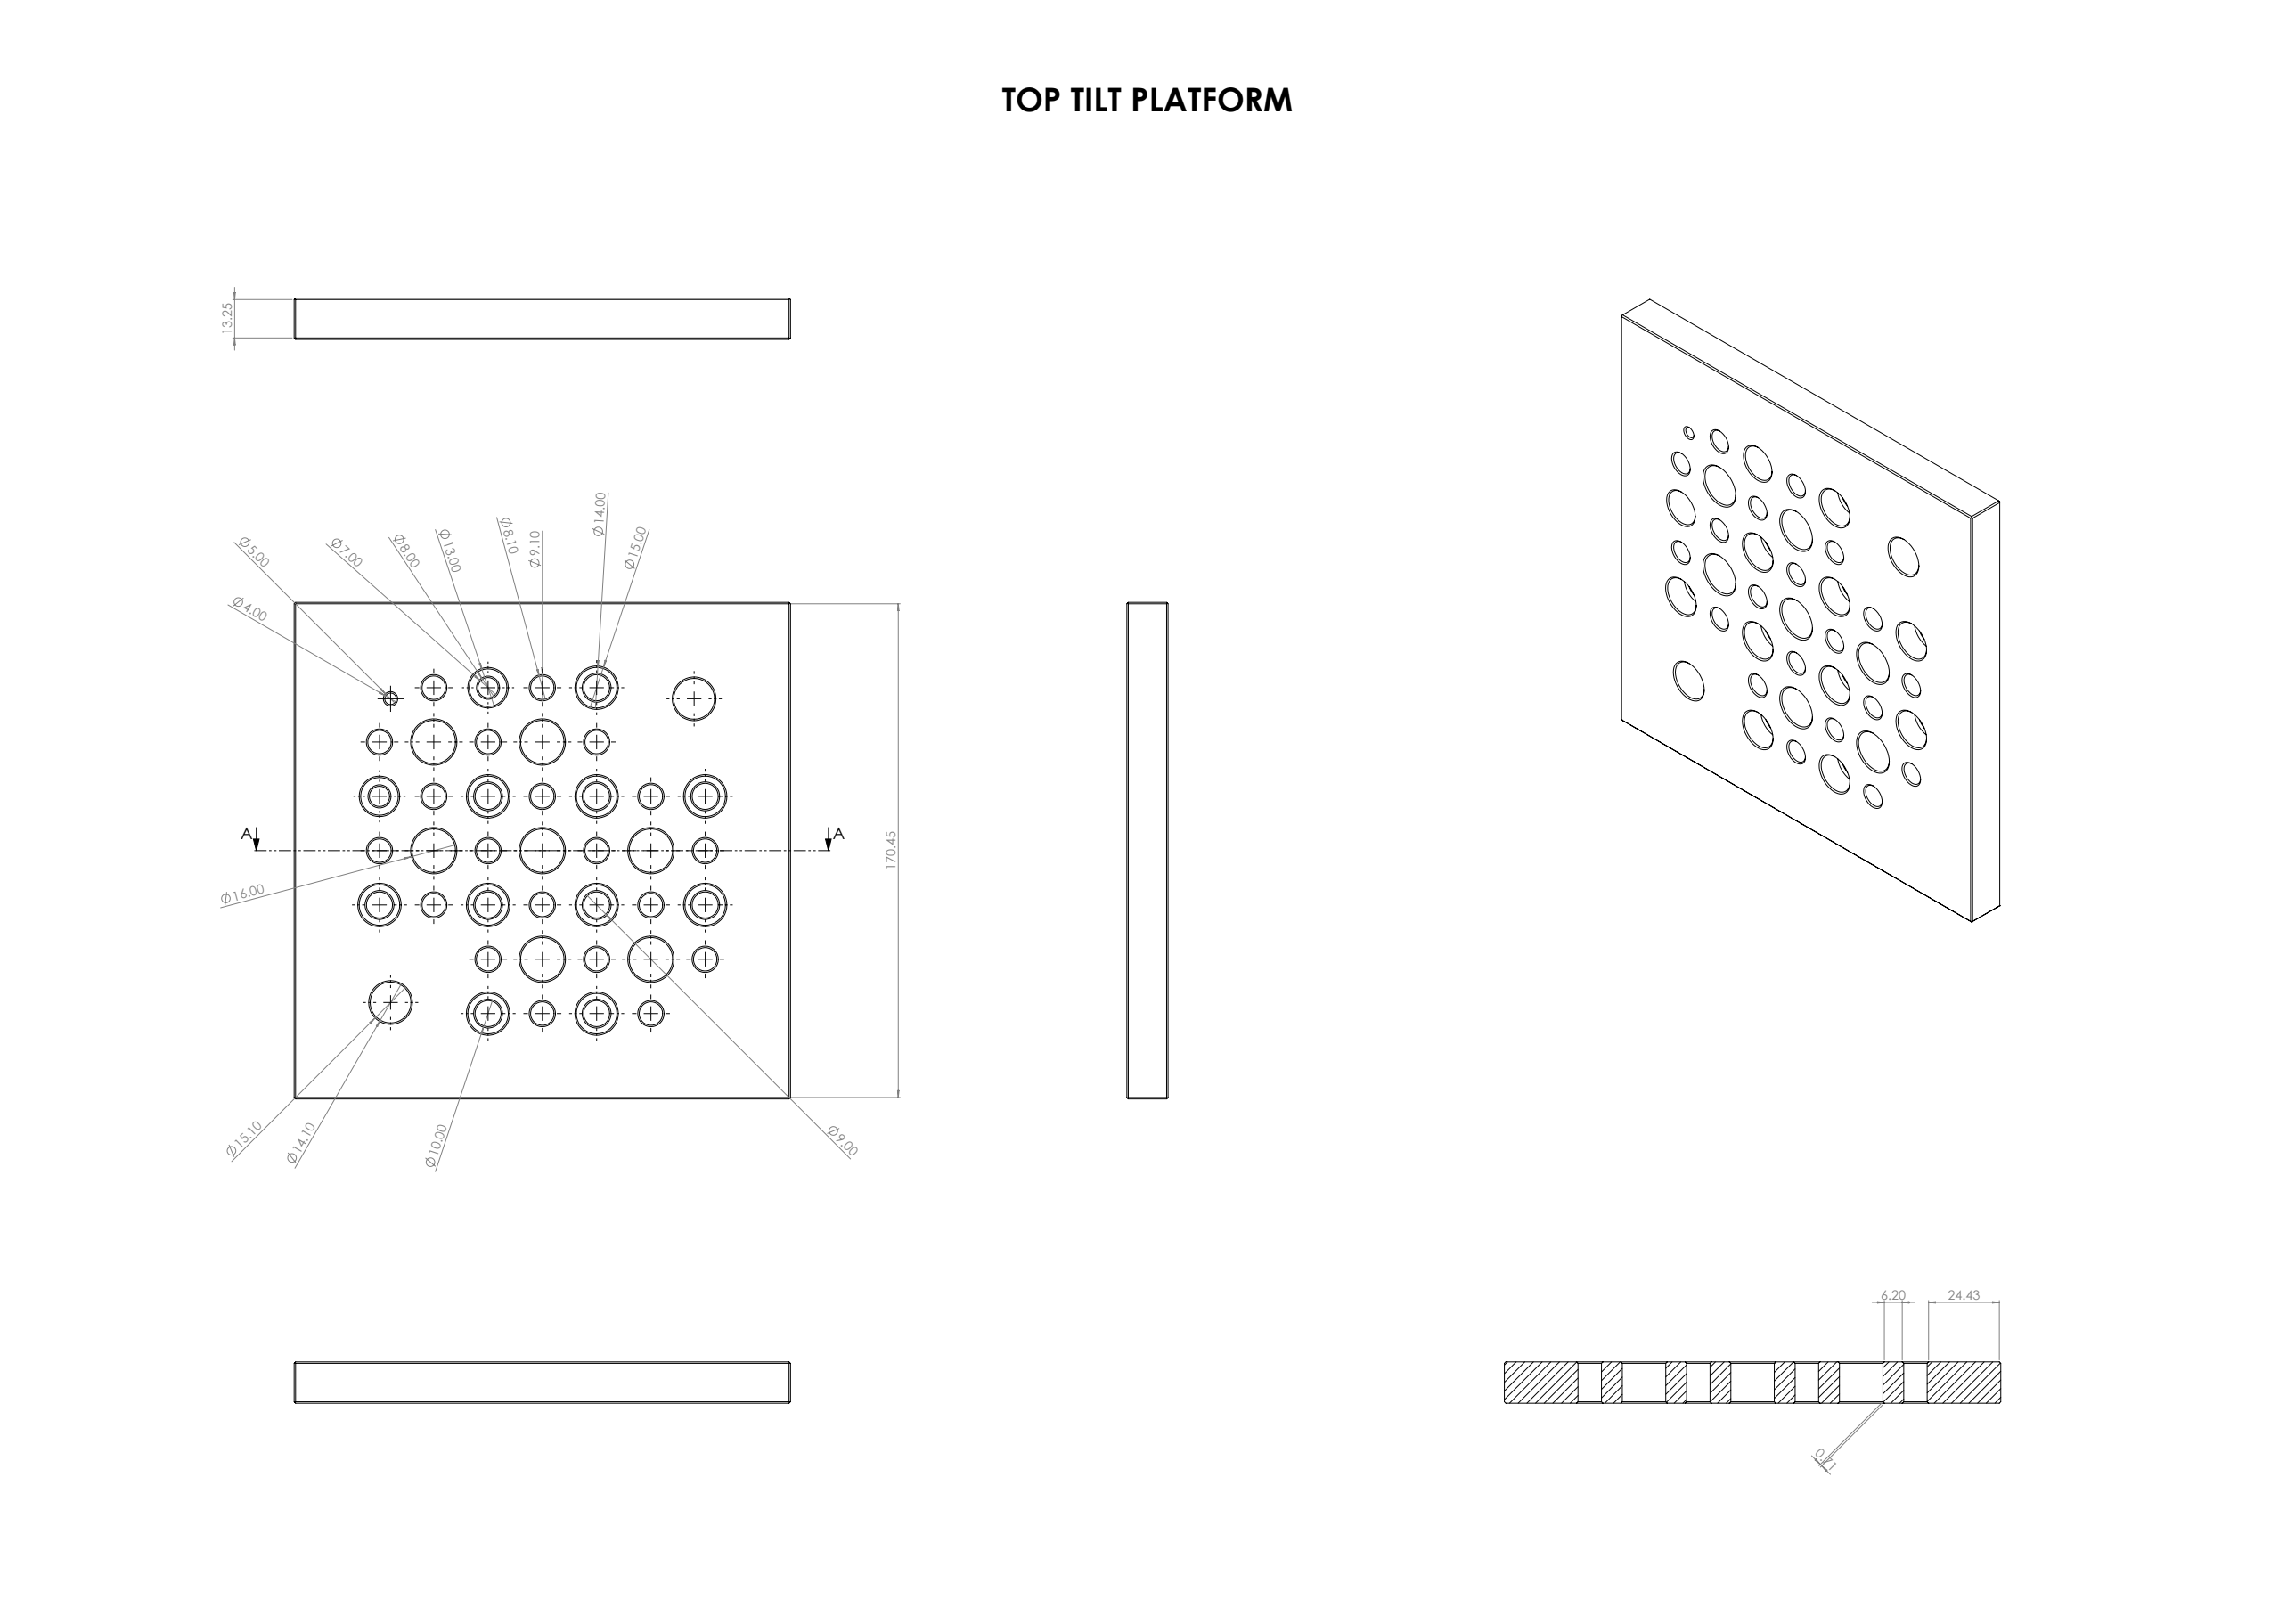
ISO-10303-21;
HEADER;
/* Generated by software containing ST-Developer
 * from STEP Tools, Inc. (www.steptools.com) 
 */

FILE_DESCRIPTION(
/* description */ (''),
/* implementation_level */ '2;1');

FILE_NAME(
/* name */ '03_Top_Tilt_Platform.step',
/* time_stamp */ '2026-10-21T01:56:51-07:00',
/* author */ (''),
/* organization */ (''),
/* preprocessor_version */ 'ST-DEVELOPER v20.2',
/* originating_system */ 'Autodesk Translation Framework v15.15.0.0',
/* authorisation */ '');

FILE_SCHEMA (('AUTOMOTIVE_DESIGN { 1 0 10303 214 3 1 1 }'));
ENDSEC;

DATA;
#10=MECHANICAL_DESIGN_GEOMETRIC_PRESENTATION_REPRESENTATION('',(#272),#82384);
#234=SHAPE_REPRESENTATION_RELATIONSHIP('SRR','None',#82468,#253);
#253=ADVANCED_BREP_SHAPE_REPRESENTATION('',(#291),#82367);
#272=STYLED_ITEM('',(#82645),#291);
#291=MANIFOLD_SOLID_BREP('Body1',#30663);
#483=CYLINDRICAL_SURFACE('',#31325,4.5);
#484=CYLINDRICAL_SURFACE('',#31332,4.5);
#485=CYLINDRICAL_SURFACE('',#31339,4.5);
#486=CYLINDRICAL_SURFACE('',#31346,4.5);
#487=CYLINDRICAL_SURFACE('',#31353,4.5);
#488=CYLINDRICAL_SURFACE('',#31360,4.5);
#489=CYLINDRICAL_SURFACE('',#31367,4.5);
#490=CYLINDRICAL_SURFACE('',#31374,4.5);
#491=CYLINDRICAL_SURFACE('',#31381,2.);
#492=CYLINDRICAL_SURFACE('',#31392,3.5);
#493=CYLINDRICAL_SURFACE('',#31399,3.5);
#494=CYLINDRICAL_SURFACE('',#31412,4.5);
#495=CYLINDRICAL_SURFACE('',#31419,4.5);
#496=CYLINDRICAL_SURFACE('',#31476,7.05);
#497=CYLINDRICAL_SURFACE('',#31480,7.05);
#498=CYLINDRICAL_SURFACE('',#31489,4.05);
#499=CYLINDRICAL_SURFACE('',#31493,4.05);
#500=CYLINDRICAL_SURFACE('',#31497,4.05);
#501=CYLINDRICAL_SURFACE('',#31501,4.05);
#502=CYLINDRICAL_SURFACE('',#31505,4.05);
#503=CYLINDRICAL_SURFACE('',#31509,4.05);
#504=CYLINDRICAL_SURFACE('',#31513,4.05);
#505=CYLINDRICAL_SURFACE('',#31517,4.05);
#506=CYLINDRICAL_SURFACE('',#31521,4.05);
#507=CYLINDRICAL_SURFACE('',#31525,4.05);
#508=CYLINDRICAL_SURFACE('',#31529,4.05);
#509=CYLINDRICAL_SURFACE('',#31533,4.05);
#510=CYLINDRICAL_SURFACE('',#31539,4.05);
#511=CYLINDRICAL_SURFACE('',#31543,4.05);
#512=CYLINDRICAL_SURFACE('',#31547,4.05);
#513=CYLINDRICAL_SURFACE('',#31551,4.05);
#514=CYLINDRICAL_SURFACE('',#31555,4.05);
#515=CYLINDRICAL_SURFACE('',#31559,4.05);
#516=CYLINDRICAL_SURFACE('',#31563,4.05);
#517=CYLINDRICAL_SURFACE('',#31567,4.05);
#518=CYLINDRICAL_SURFACE('',#31571,7.5);
#519=CYLINDRICAL_SURFACE('',#31575,7.5);
#520=CYLINDRICAL_SURFACE('',#31579,7.5);
#521=CYLINDRICAL_SURFACE('',#31583,7.5);
#522=CYLINDRICAL_SURFACE('',#31587,7.5);
#523=CYLINDRICAL_SURFACE('',#31591,7.5);
#524=CYLINDRICAL_SURFACE('',#31595,7.5);
#525=CYLINDRICAL_SURFACE('',#31652,7.);
#526=CYLINDRICAL_SURFACE('',#31655,7.);
#527=CYLINDRICAL_SURFACE('',#31658,7.);
#528=CYLINDRICAL_SURFACE('',#31661,7.);
#529=CYLINDRICAL_SURFACE('',#31664,7.);
#530=CYLINDRICAL_SURFACE('',#31667,7.);
#531=CYLINDRICAL_SURFACE('',#31670,7.);
#532=CYLINDRICAL_SURFACE('',#31673,7.);
#533=CYLINDRICAL_SURFACE('',#31676,7.);
#534=CYLINDRICAL_SURFACE('',#31679,7.);
#535=CYLINDRICAL_SURFACE('',#31704,6.5);
#536=CYLINDRICAL_SURFACE('',#31707,6.5);
#537=CYLINDRICAL_SURFACE('',#31708,4.2379);
#1196=CIRCLE('',#31323,4.5);
#1197=CIRCLE('',#31324,5.);
#1198=CIRCLE('',#31326,4.5);
#1199=CIRCLE('',#31328,7.);
#1200=CIRCLE('',#31330,4.5);
#1201=CIRCLE('',#31331,5.);
#1202=CIRCLE('',#31333,4.5);
#1203=CIRCLE('',#31335,7.);
#1204=CIRCLE('',#31337,4.5);
#1205=CIRCLE('',#31338,5.);
#1206=CIRCLE('',#31340,4.5);
#1207=CIRCLE('',#31342,7.);
#1208=CIRCLE('',#31344,4.5);
#1209=CIRCLE('',#31345,5.);
#1210=CIRCLE('',#31347,4.5);
#1211=CIRCLE('',#31349,7.);
#1212=CIRCLE('',#31351,4.5);
#1213=CIRCLE('',#31352,5.);
#1214=CIRCLE('',#31354,4.5);
#1215=CIRCLE('',#31356,7.);
#1216=CIRCLE('',#31358,4.5);
#1217=CIRCLE('',#31359,5.);
#1218=CIRCLE('',#31361,4.5);
#1219=CIRCLE('',#31363,7.);
#1220=CIRCLE('',#31365,4.5);
#1221=CIRCLE('',#31366,5.);
#1222=CIRCLE('',#31368,4.5);
#1223=CIRCLE('',#31370,7.);
#1224=CIRCLE('',#31372,4.5);
#1225=CIRCLE('',#31373,5.);
#1226=CIRCLE('',#31375,4.5);
#1227=CIRCLE('',#31377,7.);
#1228=CIRCLE('',#31379,2.);
#1229=CIRCLE('',#31380,2.5);
#1230=CIRCLE('',#31382,2.);
#1231=CIRCLE('',#31384,4.2379);
#1232=CIRCLE('',#31390,3.5);
#1233=CIRCLE('',#31391,4.);
#1234=CIRCLE('',#31393,3.5);
#1235=CIRCLE('',#31395,6.5);
#1236=CIRCLE('',#31397,3.5);
#1237=CIRCLE('',#31398,3.99999999999999);
#1238=CIRCLE('',#31400,3.5);
#1239=CIRCLE('',#31402,6.5);
#1240=CIRCLE('',#31410,4.5);
#1241=CIRCLE('',#31411,5.);
#1242=CIRCLE('',#31413,4.5);
#1243=CIRCLE('',#31415,7.);
#1244=CIRCLE('',#31417,4.5);
#1245=CIRCLE('',#31418,5.);
#1246=CIRCLE('',#31420,4.5);
#1247=CIRCLE('',#31422,7.);
#1248=CIRCLE('',#31424,5.);
#1249=CIRCLE('',#31426,5.);
#1250=CIRCLE('',#31427,5.);
#1251=CIRCLE('',#31428,5.);
#1252=CIRCLE('',#31429,5.);
#1253=CIRCLE('',#31430,7.55);
#1254=CIRCLE('',#31431,5.);
#1255=CIRCLE('',#31432,4.55);
#1256=CIRCLE('',#31433,4.55);
#1257=CIRCLE('',#31434,4.55);
#1258=CIRCLE('',#31435,4.55);
#1259=CIRCLE('',#31436,4.55);
#1260=CIRCLE('',#31437,4.55);
#1261=CIRCLE('',#31438,3.99999999999999);
#1262=CIRCLE('',#31439,4.55);
#1263=CIRCLE('',#31440,4.55);
#1264=CIRCLE('',#31441,4.55);
#1265=CIRCLE('',#31442,4.55);
#1266=CIRCLE('',#31443,8.);
#1267=CIRCLE('',#31444,8.);
#1268=CIRCLE('',#31445,8.);
#1269=CIRCLE('',#31446,8.);
#1270=CIRCLE('',#31447,4.2379);
#1271=CIRCLE('',#31448,8.);
#1272=CIRCLE('',#31449,8.);
#1273=CIRCLE('',#31450,8.);
#1274=CIRCLE('',#31451,4.55);
#1275=CIRCLE('',#31452,4.55);
#1276=CIRCLE('',#31453,4.55);
#1277=CIRCLE('',#31454,4.55);
#1278=CIRCLE('',#31455,4.);
#1279=CIRCLE('',#31456,4.55);
#1280=CIRCLE('',#31457,4.55);
#1281=CIRCLE('',#31458,4.55);
#1282=CIRCLE('',#31459,4.55);
#1283=CIRCLE('',#31460,4.55);
#1284=CIRCLE('',#31461,4.55);
#1285=CIRCLE('',#31462,5.);
#1286=CIRCLE('',#31463,7.55);
#1287=CIRCLE('',#31464,5.);
#1288=CIRCLE('',#31465,5.);
#1289=CIRCLE('',#31466,5.);
#1290=CIRCLE('',#31475,7.05);
#1291=CIRCLE('',#31477,7.05);
#1292=CIRCLE('',#31479,7.05);
#1293=CIRCLE('',#31481,7.05);
#1294=CIRCLE('',#31488,4.05);
#1295=CIRCLE('',#31490,4.05);
#1296=CIRCLE('',#31492,4.05);
#1297=CIRCLE('',#31494,4.05);
#1298=CIRCLE('',#31496,4.05);
#1299=CIRCLE('',#31498,4.05);
#1300=CIRCLE('',#31500,4.05);
#1301=CIRCLE('',#31502,4.05);
#1302=CIRCLE('',#31504,4.05);
#1303=CIRCLE('',#31506,4.05);
#1304=CIRCLE('',#31508,4.05);
#1305=CIRCLE('',#31510,4.05);
#1306=CIRCLE('',#31512,4.05);
#1307=CIRCLE('',#31514,4.05);
#1308=CIRCLE('',#31516,4.05);
#1309=CIRCLE('',#31518,4.05);
#1310=CIRCLE('',#31520,4.05);
#1311=CIRCLE('',#31522,4.05);
#1312=CIRCLE('',#31524,4.05);
#1313=CIRCLE('',#31526,4.05);
#1314=CIRCLE('',#31528,4.05);
#1315=CIRCLE('',#31530,4.05);
#1316=CIRCLE('',#31532,4.05);
#1317=CIRCLE('',#31534,4.05);
#1318=CIRCLE('',#31538,4.05);
#1319=CIRCLE('',#31540,4.05);
#1320=CIRCLE('',#31542,4.05);
#1321=CIRCLE('',#31544,4.05);
#1322=CIRCLE('',#31546,4.05);
#1323=CIRCLE('',#31548,4.05);
#1324=CIRCLE('',#31550,4.05);
#1325=CIRCLE('',#31552,4.05);
#1326=CIRCLE('',#31554,4.05);
#1327=CIRCLE('',#31556,4.05);
#1328=CIRCLE('',#31558,4.05);
#1329=CIRCLE('',#31560,4.05);
#1330=CIRCLE('',#31562,4.05);
#1331=CIRCLE('',#31564,4.05);
#1332=CIRCLE('',#31566,4.05);
#1333=CIRCLE('',#31568,4.05);
#1334=CIRCLE('',#31570,7.5);
#1335=CIRCLE('',#31572,7.5);
#1336=CIRCLE('',#31574,7.5);
#1337=CIRCLE('',#31576,7.5);
#1338=CIRCLE('',#31578,7.5);
#1339=CIRCLE('',#31580,7.5);
#1340=CIRCLE('',#31582,7.5);
#1341=CIRCLE('',#31584,7.5);
#1342=CIRCLE('',#31586,7.5);
#1343=CIRCLE('',#31588,7.5);
#1344=CIRCLE('',#31590,7.5);
#1345=CIRCLE('',#31592,7.5);
#1346=CIRCLE('',#31594,7.5);
#1347=CIRCLE('',#31596,7.5);
#1348=CIRCLE('',#31600,2.5);
#1349=CIRCLE('',#31601,8.);
#1350=CIRCLE('',#31602,8.);
#1351=CIRCLE('',#31603,8.);
#1352=CIRCLE('',#31604,7.5);
#1353=CIRCLE('',#31605,7.5);
#1354=CIRCLE('',#31606,7.5);
#1355=CIRCLE('',#31607,7.5);
#1356=CIRCLE('',#31608,7.5);
#1357=CIRCLE('',#31609,4.55);
#1358=CIRCLE('',#31610,4.55);
#1359=CIRCLE('',#31611,4.55);
#1360=CIRCLE('',#31612,4.55);
#1361=CIRCLE('',#31613,4.55);
#1362=CIRCLE('',#31614,4.55);
#1363=CIRCLE('',#31615,4.55);
#1364=CIRCLE('',#31616,4.55);
#1365=CIRCLE('',#31617,4.55);
#1366=CIRCLE('',#31618,4.55);
#1367=CIRCLE('',#31619,7.55);
#1368=CIRCLE('',#31620,7.);
#1369=CIRCLE('',#31621,7.);
#1370=CIRCLE('',#31622,7.55);
#1371=CIRCLE('',#31623,4.55);
#1372=CIRCLE('',#31624,4.55);
#1373=CIRCLE('',#31625,4.55);
#1374=CIRCLE('',#31626,4.55);
#1375=CIRCLE('',#31627,4.55);
#1376=CIRCLE('',#31628,4.55);
#1377=CIRCLE('',#31629,4.55);
#1378=CIRCLE('',#31630,4.55);
#1379=CIRCLE('',#31631,4.55);
#1380=CIRCLE('',#31632,4.55);
#1381=CIRCLE('',#31633,7.5);
#1382=CIRCLE('',#31634,7.5);
#1383=CIRCLE('',#31635,7.5);
#1384=CIRCLE('',#31636,7.5);
#1385=CIRCLE('',#31637,7.5);
#1386=CIRCLE('',#31638,8.);
#1387=CIRCLE('',#31639,8.);
#1388=CIRCLE('',#31640,8.);
#1389=CIRCLE('',#31641,8.);
#1390=CIRCLE('',#31651,7.);
#1391=CIRCLE('',#31654,7.);
#1392=CIRCLE('',#31657,7.);
#1393=CIRCLE('',#31660,7.);
#1394=CIRCLE('',#31663,7.);
#1395=CIRCLE('',#31666,7.);
#1396=CIRCLE('',#31669,7.);
#1397=CIRCLE('',#31672,7.);
#1398=CIRCLE('',#31675,7.);
#1399=CIRCLE('',#31678,7.);
#1400=CIRCLE('',#31703,6.5);
#1401=CIRCLE('',#31706,6.5);
#1933=CONICAL_SURFACE('',#31322,4.75,0.785398163397448);
#1934=CONICAL_SURFACE('',#31329,4.75,0.785398163397448);
#1935=CONICAL_SURFACE('',#31336,4.75,0.785398163397451);
#1936=CONICAL_SURFACE('',#31343,4.75,0.785398163397451);
#1937=CONICAL_SURFACE('',#31350,4.75,0.785398163397451);
#1938=CONICAL_SURFACE('',#31357,4.75,0.785398163397448);
#1939=CONICAL_SURFACE('',#31364,4.75,0.785398163397448);
#1940=CONICAL_SURFACE('',#31371,4.75,0.785398163397448);
#1941=CONICAL_SURFACE('',#31378,2.25,0.785398163397448);
#1942=CONICAL_SURFACE('',#31389,3.75,0.785398163397451);
#1943=CONICAL_SURFACE('',#31396,3.75,0.785398163397448);
#1944=CONICAL_SURFACE('',#31409,4.75,0.785398163397448);
#1945=CONICAL_SURFACE('',#31416,4.75,0.785398163397448);
#1946=CONICAL_SURFACE('',#31423,4.75,0.785398163397448);
#1947=CONICAL_SURFACE('',#31467,4.75,0.785398163397448);
#1948=CONICAL_SURFACE('',#31468,4.75,0.785398163397451);
#1949=CONICAL_SURFACE('',#31469,4.75,0.785398163397451);
#1950=CONICAL_SURFACE('',#31470,4.75,0.785398163397451);
#1951=CONICAL_SURFACE('',#31471,4.75,0.785398163397448);
#1952=CONICAL_SURFACE('',#31472,4.75,0.785398163397448);
#1953=CONICAL_SURFACE('',#31473,4.75,0.785398163397448);
#1954=CONICAL_SURFACE('',#31474,7.3,0.785398163397448);
#1955=CONICAL_SURFACE('',#31478,7.3,0.785398163397448);
#1956=CONICAL_SURFACE('',#31482,4.75,0.785398163397448);
#1957=CONICAL_SURFACE('',#31483,4.75,0.785398163397448);
#1958=CONICAL_SURFACE('',#31487,4.3,0.785398163397448);
#1959=CONICAL_SURFACE('',#31491,4.3,0.785398163397448);
#1960=CONICAL_SURFACE('',#31495,4.3,0.785398163397448);
#1961=CONICAL_SURFACE('',#31499,4.3,0.785398163397448);
#1962=CONICAL_SURFACE('',#31503,4.3,0.785398163397451);
#1963=CONICAL_SURFACE('',#31507,4.3,0.785398163397451);
#1964=CONICAL_SURFACE('',#31511,4.3,0.78539816339745);
#1965=CONICAL_SURFACE('',#31515,4.3,0.78539816339745);
#1966=CONICAL_SURFACE('',#31519,4.3,0.785398163397448);
#1967=CONICAL_SURFACE('',#31523,4.3,0.785398163397448);
#1968=CONICAL_SURFACE('',#31527,4.3,0.785398163397448);
#1969=CONICAL_SURFACE('',#31531,4.3,0.785398163397448);
#1970=CONICAL_SURFACE('',#31535,3.75,0.785398163397448);
#1971=CONICAL_SURFACE('',#31536,3.75,0.785398163397451);
#1972=CONICAL_SURFACE('',#31537,4.3,0.785398163397451);
#1973=CONICAL_SURFACE('',#31541,4.3,0.78539816339745);
#1974=CONICAL_SURFACE('',#31545,4.3,0.785398163397448);
#1975=CONICAL_SURFACE('',#31549,4.3,0.78539816339745);
#1976=CONICAL_SURFACE('',#31553,4.3,0.785398163397448);
#1977=CONICAL_SURFACE('',#31557,4.3,0.785398163397448);
#1978=CONICAL_SURFACE('',#31561,4.3,0.785398163397448);
#1979=CONICAL_SURFACE('',#31565,4.3,0.785398163397448);
#1980=CONICAL_SURFACE('',#31569,7.75,0.785398163397448);
#1981=CONICAL_SURFACE('',#31573,7.75,0.785398163397448);
#1982=CONICAL_SURFACE('',#31577,7.75,0.785398163397451);
#1983=CONICAL_SURFACE('',#31581,7.75,0.785398163397448);
#1984=CONICAL_SURFACE('',#31585,7.75,0.785398163397451);
#1985=CONICAL_SURFACE('',#31589,7.75,0.785398163397451);
#1986=CONICAL_SURFACE('',#31593,7.75,0.785398163397448);
#1987=CONICAL_SURFACE('',#31642,2.25,0.785398163397448);
#1988=CONICAL_SURFACE('',#31643,7.75,0.785398163397448);
#1989=CONICAL_SURFACE('',#31644,7.75,0.785398163397451);
#1990=CONICAL_SURFACE('',#31645,7.75,0.785398163397451);
#1991=CONICAL_SURFACE('',#31646,7.75,0.785398163397448);
#1992=CONICAL_SURFACE('',#31647,7.75,0.785398163397451);
#1993=CONICAL_SURFACE('',#31648,7.75,0.785398163397448);
#1994=CONICAL_SURFACE('',#31649,7.75,0.785398163397448);
#1995=CONICAL_SURFACE('',#31650,7.25,0.785398163397448);
#1996=CONICAL_SURFACE('',#31653,7.25,0.785398163397448);
#1997=CONICAL_SURFACE('',#31656,7.25,0.785398163397448);
#1998=CONICAL_SURFACE('',#31659,7.25,0.785398163397448);
#1999=CONICAL_SURFACE('',#31662,7.25,0.785398163397451);
#2000=CONICAL_SURFACE('',#31665,7.25,0.785398163397451);
#2001=CONICAL_SURFACE('',#31668,7.25,0.785398163397451);
#2002=CONICAL_SURFACE('',#31671,7.25,0.785398163397448);
#2003=CONICAL_SURFACE('',#31674,7.25,0.785398163397448);
#2004=CONICAL_SURFACE('',#31677,7.25,0.785398163397448);
#2005=CONICAL_SURFACE('',#31680,4.3,0.785398163397448);
#2006=CONICAL_SURFACE('',#31681,4.3,0.785398163397448);
#2007=CONICAL_SURFACE('',#31682,4.3,0.785398163397448);
#2008=CONICAL_SURFACE('',#31683,4.3,0.785398163397448);
#2009=CONICAL_SURFACE('',#31684,4.3,0.78539816339745);
#2010=CONICAL_SURFACE('',#31685,4.3,0.785398163397448);
#2011=CONICAL_SURFACE('',#31686,4.3,0.78539816339745);
#2012=CONICAL_SURFACE('',#31687,4.3,0.785398163397451);
#2013=CONICAL_SURFACE('',#31688,4.3,0.785398163397448);
#2014=CONICAL_SURFACE('',#31689,4.3,0.785398163397448);
#2015=CONICAL_SURFACE('',#31690,4.3,0.785398163397448);
#2016=CONICAL_SURFACE('',#31691,4.3,0.785398163397448);
#2017=CONICAL_SURFACE('',#31692,4.3,0.785398163397451);
#2018=CONICAL_SURFACE('',#31693,4.3,0.785398163397451);
#2019=CONICAL_SURFACE('',#31694,4.3,0.78539816339745);
#2020=CONICAL_SURFACE('',#31695,4.3,0.78539816339745);
#2021=CONICAL_SURFACE('',#31696,4.3,0.785398163397448);
#2022=CONICAL_SURFACE('',#31697,4.3,0.785398163397448);
#2023=CONICAL_SURFACE('',#31698,4.3,0.785398163397448);
#2024=CONICAL_SURFACE('',#31699,4.3,0.785398163397448);
#2025=CONICAL_SURFACE('',#31700,7.3,0.785398163397448);
#2026=CONICAL_SURFACE('',#31701,7.3,0.785398163397448);
#2027=CONICAL_SURFACE('',#31702,6.75,0.785398163397448);
#2028=CONICAL_SURFACE('',#31705,6.75,0.785398163397451);
#3337=FACE_BOUND('',#5767,.T.);
#3338=FACE_BOUND('',#5771,.T.);
#3339=FACE_BOUND('',#5775,.T.);
#3340=FACE_BOUND('',#5779,.T.);
#3341=FACE_BOUND('',#5783,.T.);
#3342=FACE_BOUND('',#5787,.T.);
#3343=FACE_BOUND('',#5791,.T.);
#3344=FACE_BOUND('',#5795,.T.);
#3345=FACE_BOUND('',#5799,.T.);
#3346=FACE_BOUND('',#5807,.T.);
#3347=FACE_BOUND('',#5811,.T.);
#3348=FACE_BOUND('',#5821,.T.);
#3349=FACE_BOUND('',#5825,.T.);
#3350=FACE_BOUND('',#5828,.T.);
#3351=FACE_BOUND('',#5829,.T.);
#3352=FACE_BOUND('',#5830,.T.);
#3353=FACE_BOUND('',#5831,.T.);
#3354=FACE_BOUND('',#5832,.T.);
#3355=FACE_BOUND('',#5833,.T.);
#3356=FACE_BOUND('',#5834,.T.);
#3357=FACE_BOUND('',#5835,.T.);
#3358=FACE_BOUND('',#5836,.T.);
#3359=FACE_BOUND('',#5837,.T.);
#3360=FACE_BOUND('',#5838,.T.);
#3361=FACE_BOUND('',#5839,.T.);
#3362=FACE_BOUND('',#5840,.T.);
#3363=FACE_BOUND('',#5841,.T.);
#3364=FACE_BOUND('',#5842,.T.);
#3365=FACE_BOUND('',#5843,.T.);
#3366=FACE_BOUND('',#5844,.T.);
#3367=FACE_BOUND('',#5845,.T.);
#3368=FACE_BOUND('',#5846,.T.);
#3369=FACE_BOUND('',#5847,.T.);
#3370=FACE_BOUND('',#5848,.T.);
#3371=FACE_BOUND('',#5849,.T.);
#3372=FACE_BOUND('',#5850,.T.);
#3373=FACE_BOUND('',#5851,.T.);
#3374=FACE_BOUND('',#5852,.T.);
#3375=FACE_BOUND('',#5853,.T.);
#3376=FACE_BOUND('',#5854,.T.);
#3377=FACE_BOUND('',#5855,.T.);
#3378=FACE_BOUND('',#5856,.T.);
#3379=FACE_BOUND('',#5857,.T.);
#3380=FACE_BOUND('',#5858,.T.);
#3381=FACE_BOUND('',#5859,.T.);
#3382=FACE_BOUND('',#5860,.T.);
#3383=FACE_BOUND('',#5861,.T.);
#3384=FACE_BOUND('',#5862,.T.);
#3385=FACE_BOUND('',#5863,.T.);
#3386=FACE_BOUND('',#5864,.T.);
#3387=FACE_BOUND('',#5865,.T.);
#3388=FACE_BOUND('',#5866,.T.);
#3389=FACE_BOUND('',#5867,.T.);
#3390=FACE_BOUND('',#5868,.T.);
#3391=FACE_BOUND('',#5869,.T.);
#3392=FACE_BOUND('',#5945,.T.);
#3393=FACE_BOUND('',#5946,.T.);
#3394=FACE_BOUND('',#5947,.T.);
#3395=FACE_BOUND('',#5948,.T.);
#3396=FACE_BOUND('',#5949,.T.);
#3397=FACE_BOUND('',#5950,.T.);
#3398=FACE_BOUND('',#5951,.T.);
#3399=FACE_BOUND('',#5952,.T.);
#3400=FACE_BOUND('',#5953,.T.);
#3401=FACE_BOUND('',#5954,.T.);
#3402=FACE_BOUND('',#5955,.T.);
#3403=FACE_BOUND('',#5956,.T.);
#3404=FACE_BOUND('',#5957,.T.);
#3405=FACE_BOUND('',#5958,.T.);
#3406=FACE_BOUND('',#5959,.T.);
#3407=FACE_BOUND('',#5960,.T.);
#3408=FACE_BOUND('',#5961,.T.);
#3409=FACE_BOUND('',#5962,.T.);
#3410=FACE_BOUND('',#5963,.T.);
#3411=FACE_BOUND('',#5964,.T.);
#3412=FACE_BOUND('',#5965,.T.);
#3413=FACE_BOUND('',#5966,.T.);
#3414=FACE_BOUND('',#5967,.T.);
#3415=FACE_BOUND('',#5968,.T.);
#3416=FACE_BOUND('',#5969,.T.);
#3417=FACE_BOUND('',#5970,.T.);
#3418=FACE_BOUND('',#5971,.T.);
#3419=FACE_BOUND('',#5972,.T.);
#3420=FACE_BOUND('',#5973,.T.);
#3421=FACE_BOUND('',#5974,.T.);
#3422=FACE_BOUND('',#5975,.T.);
#3423=FACE_BOUND('',#5976,.T.);
#3424=FACE_BOUND('',#5977,.T.);
#3425=FACE_BOUND('',#5978,.T.);
#3426=FACE_BOUND('',#5979,.T.);
#3427=FACE_BOUND('',#5980,.T.);
#3428=FACE_BOUND('',#5981,.T.);
#3429=FACE_BOUND('',#5982,.T.);
#3430=FACE_BOUND('',#5983,.T.);
#3431=FACE_BOUND('',#5984,.T.);
#3432=FACE_BOUND('',#5985,.T.);
#3433=FACE_BOUND('',#5986,.T.);
#3955=FACE_OUTER_BOUND('',#5764,.T.);
#3956=FACE_OUTER_BOUND('',#5765,.T.);
#3957=FACE_OUTER_BOUND('',#5766,.T.);
#3958=FACE_OUTER_BOUND('',#5768,.T.);
#3959=FACE_OUTER_BOUND('',#5769,.T.);
#3960=FACE_OUTER_BOUND('',#5770,.T.);
#3961=FACE_OUTER_BOUND('',#5772,.T.);
#3962=FACE_OUTER_BOUND('',#5773,.T.);
#3963=FACE_OUTER_BOUND('',#5774,.T.);
#3964=FACE_OUTER_BOUND('',#5776,.T.);
#3965=FACE_OUTER_BOUND('',#5777,.T.);
#3966=FACE_OUTER_BOUND('',#5778,.T.);
#3967=FACE_OUTER_BOUND('',#5780,.T.);
#3968=FACE_OUTER_BOUND('',#5781,.T.);
#3969=FACE_OUTER_BOUND('',#5782,.T.);
#3970=FACE_OUTER_BOUND('',#5784,.T.);
#3971=FACE_OUTER_BOUND('',#5785,.T.);
#3972=FACE_OUTER_BOUND('',#5786,.T.);
#3973=FACE_OUTER_BOUND('',#5788,.T.);
#3974=FACE_OUTER_BOUND('',#5789,.T.);
#3975=FACE_OUTER_BOUND('',#5790,.T.);
#3976=FACE_OUTER_BOUND('',#5792,.T.);
#3977=FACE_OUTER_BOUND('',#5793,.T.);
#3978=FACE_OUTER_BOUND('',#5794,.T.);
#3979=FACE_OUTER_BOUND('',#5796,.T.);
#3980=FACE_OUTER_BOUND('',#5797,.T.);
#3981=FACE_OUTER_BOUND('',#5798,.T.);
#3982=FACE_OUTER_BOUND('',#5800,.T.);
#3983=FACE_OUTER_BOUND('',#5801,.T.);
#3984=FACE_OUTER_BOUND('',#5802,.T.);
#3985=FACE_OUTER_BOUND('',#5803,.T.);
#3986=FACE_OUTER_BOUND('',#5804,.T.);
#3987=FACE_OUTER_BOUND('',#5805,.T.);
#3988=FACE_OUTER_BOUND('',#5806,.T.);
#3989=FACE_OUTER_BOUND('',#5808,.T.);
#3990=FACE_OUTER_BOUND('',#5809,.T.);
#3991=FACE_OUTER_BOUND('',#5810,.T.);
#3992=FACE_OUTER_BOUND('',#5812,.T.);
#3993=FACE_OUTER_BOUND('',#5813,.T.);
#3994=FACE_OUTER_BOUND('',#5814,.T.);
#3995=FACE_OUTER_BOUND('',#5815,.T.);
#3996=FACE_OUTER_BOUND('',#5816,.T.);
#3997=FACE_OUTER_BOUND('',#5817,.T.);
#3998=FACE_OUTER_BOUND('',#5818,.T.);
#3999=FACE_OUTER_BOUND('',#5819,.T.);
#4000=FACE_OUTER_BOUND('',#5820,.T.);
#4001=FACE_OUTER_BOUND('',#5822,.T.);
#4002=FACE_OUTER_BOUND('',#5823,.T.);
#4003=FACE_OUTER_BOUND('',#5824,.T.);
#4004=FACE_OUTER_BOUND('',#5826,.T.);
#4005=FACE_OUTER_BOUND('',#5827,.T.);
#4006=FACE_OUTER_BOUND('',#5870,.T.);
#4007=FACE_OUTER_BOUND('',#5871,.T.);
#4008=FACE_OUTER_BOUND('',#5872,.T.);
#4009=FACE_OUTER_BOUND('',#5873,.T.);
#4010=FACE_OUTER_BOUND('',#5874,.T.);
#4011=FACE_OUTER_BOUND('',#5875,.T.);
#4012=FACE_OUTER_BOUND('',#5876,.T.);
#4013=FACE_OUTER_BOUND('',#5877,.T.);
#4014=FACE_OUTER_BOUND('',#5878,.T.);
#4015=FACE_OUTER_BOUND('',#5879,.T.);
#4016=FACE_OUTER_BOUND('',#5880,.T.);
#4017=FACE_OUTER_BOUND('',#5881,.T.);
#4018=FACE_OUTER_BOUND('',#5882,.T.);
#4019=FACE_OUTER_BOUND('',#5883,.T.);
#4020=FACE_OUTER_BOUND('',#5884,.T.);
#4021=FACE_OUTER_BOUND('',#5885,.T.);
#4022=FACE_OUTER_BOUND('',#5886,.T.);
#4023=FACE_OUTER_BOUND('',#5887,.T.);
#4024=FACE_OUTER_BOUND('',#5888,.T.);
#4025=FACE_OUTER_BOUND('',#5889,.T.);
#4026=FACE_OUTER_BOUND('',#5890,.T.);
#4027=FACE_OUTER_BOUND('',#5891,.T.);
#4028=FACE_OUTER_BOUND('',#5892,.T.);
#4029=FACE_OUTER_BOUND('',#5893,.T.);
#4030=FACE_OUTER_BOUND('',#5894,.T.);
#4031=FACE_OUTER_BOUND('',#5895,.T.);
#4032=FACE_OUTER_BOUND('',#5896,.T.);
#4033=FACE_OUTER_BOUND('',#5897,.T.);
#4034=FACE_OUTER_BOUND('',#5898,.T.);
#4035=FACE_OUTER_BOUND('',#5899,.T.);
#4036=FACE_OUTER_BOUND('',#5900,.T.);
#4037=FACE_OUTER_BOUND('',#5901,.T.);
#4038=FACE_OUTER_BOUND('',#5902,.T.);
#4039=FACE_OUTER_BOUND('',#5903,.T.);
#4040=FACE_OUTER_BOUND('',#5904,.T.);
#4041=FACE_OUTER_BOUND('',#5905,.T.);
#4042=FACE_OUTER_BOUND('',#5906,.T.);
#4043=FACE_OUTER_BOUND('',#5907,.T.);
#4044=FACE_OUTER_BOUND('',#5908,.T.);
#4045=FACE_OUTER_BOUND('',#5909,.T.);
#4046=FACE_OUTER_BOUND('',#5910,.T.);
#4047=FACE_OUTER_BOUND('',#5911,.T.);
#4048=FACE_OUTER_BOUND('',#5912,.T.);
#4049=FACE_OUTER_BOUND('',#5913,.T.);
#4050=FACE_OUTER_BOUND('',#5914,.T.);
#4051=FACE_OUTER_BOUND('',#5915,.T.);
#4052=FACE_OUTER_BOUND('',#5916,.T.);
#4053=FACE_OUTER_BOUND('',#5917,.T.);
#4054=FACE_OUTER_BOUND('',#5918,.T.);
#4055=FACE_OUTER_BOUND('',#5919,.T.);
#4056=FACE_OUTER_BOUND('',#5920,.T.);
#4057=FACE_OUTER_BOUND('',#5921,.T.);
#4058=FACE_OUTER_BOUND('',#5922,.T.);
#4059=FACE_OUTER_BOUND('',#5923,.T.);
#4060=FACE_OUTER_BOUND('',#5924,.T.);
#4061=FACE_OUTER_BOUND('',#5925,.T.);
#4062=FACE_OUTER_BOUND('',#5926,.T.);
#4063=FACE_OUTER_BOUND('',#5927,.T.);
#4064=FACE_OUTER_BOUND('',#5928,.T.);
#4065=FACE_OUTER_BOUND('',#5929,.T.);
#4066=FACE_OUTER_BOUND('',#5930,.T.);
#4067=FACE_OUTER_BOUND('',#5931,.T.);
#4068=FACE_OUTER_BOUND('',#5932,.T.);
#4069=FACE_OUTER_BOUND('',#5933,.T.);
#4070=FACE_OUTER_BOUND('',#5934,.T.);
#4071=FACE_OUTER_BOUND('',#5935,.T.);
#4072=FACE_OUTER_BOUND('',#5936,.T.);
#4073=FACE_OUTER_BOUND('',#5937,.T.);
#4074=FACE_OUTER_BOUND('',#5938,.T.);
#4075=FACE_OUTER_BOUND('',#5939,.T.);
#4076=FACE_OUTER_BOUND('',#5940,.T.);
#4077=FACE_OUTER_BOUND('',#5941,.T.);
#4078=FACE_OUTER_BOUND('',#5942,.T.);
#4079=FACE_OUTER_BOUND('',#5943,.T.);
#4080=FACE_OUTER_BOUND('',#5944,.T.);
#4081=FACE_OUTER_BOUND('',#5987,.T.);
#4082=FACE_OUTER_BOUND('',#5988,.T.);
#4083=FACE_OUTER_BOUND('',#5989,.T.);
#4084=FACE_OUTER_BOUND('',#5990,.T.);
#4085=FACE_OUTER_BOUND('',#5991,.T.);
#4086=FACE_OUTER_BOUND('',#5992,.T.);
#4087=FACE_OUTER_BOUND('',#5993,.T.);
#4088=FACE_OUTER_BOUND('',#5994,.T.);
#4089=FACE_OUTER_BOUND('',#5995,.T.);
#4090=FACE_OUTER_BOUND('',#5996,.T.);
#4091=FACE_OUTER_BOUND('',#5997,.T.);
#4092=FACE_OUTER_BOUND('',#5998,.T.);
#4093=FACE_OUTER_BOUND('',#5999,.T.);
#4094=FACE_OUTER_BOUND('',#6000,.T.);
#4095=FACE_OUTER_BOUND('',#6001,.T.);
#4096=FACE_OUTER_BOUND('',#6002,.T.);
#4097=FACE_OUTER_BOUND('',#6003,.T.);
#4098=FACE_OUTER_BOUND('',#6004,.T.);
#4099=FACE_OUTER_BOUND('',#6005,.T.);
#4100=FACE_OUTER_BOUND('',#6006,.T.);
#4101=FACE_OUTER_BOUND('',#6007,.T.);
#4102=FACE_OUTER_BOUND('',#6008,.T.);
#4103=FACE_OUTER_BOUND('',#6009,.T.);
#4104=FACE_OUTER_BOUND('',#6010,.T.);
#4105=FACE_OUTER_BOUND('',#6011,.T.);
#4106=FACE_OUTER_BOUND('',#6012,.T.);
#4107=FACE_OUTER_BOUND('',#6013,.T.);
#4108=FACE_OUTER_BOUND('',#6014,.T.);
#4109=FACE_OUTER_BOUND('',#6015,.T.);
#4110=FACE_OUTER_BOUND('',#6016,.T.);
#4111=FACE_OUTER_BOUND('',#6017,.T.);
#4112=FACE_OUTER_BOUND('',#6018,.T.);
#4113=FACE_OUTER_BOUND('',#6019,.T.);
#4114=FACE_OUTER_BOUND('',#6020,.T.);
#4115=FACE_OUTER_BOUND('',#6021,.T.);
#4116=FACE_OUTER_BOUND('',#6022,.T.);
#4117=FACE_OUTER_BOUND('',#6023,.T.);
#4118=FACE_OUTER_BOUND('',#6024,.T.);
#4119=FACE_OUTER_BOUND('',#6025,.T.);
#4120=FACE_OUTER_BOUND('',#6026,.T.);
#4121=FACE_OUTER_BOUND('',#6027,.T.);
#4122=FACE_OUTER_BOUND('',#6028,.T.);
#4123=FACE_OUTER_BOUND('',#6029,.T.);
#4124=FACE_OUTER_BOUND('',#6030,.T.);
#4125=FACE_OUTER_BOUND('',#6031,.T.);
#4126=FACE_OUTER_BOUND('',#6032,.T.);
#4127=FACE_OUTER_BOUND('',#6033,.T.);
#4128=FACE_OUTER_BOUND('',#6034,.T.);
#4129=FACE_OUTER_BOUND('',#6035,.T.);
#4130=FACE_OUTER_BOUND('',#6036,.T.);
#4131=FACE_OUTER_BOUND('',#6037,.T.);
#4132=FACE_OUTER_BOUND('',#6038,.T.);
#4133=FACE_OUTER_BOUND('',#6039,.T.);
#4134=FACE_OUTER_BOUND('',#6040,.T.);
#4135=FACE_OUTER_BOUND('',#6041,.T.);
#4136=FACE_OUTER_BOUND('',#6042,.T.);
#5764=EDGE_LOOP('',(#21119,#21120,#21121,#21122));
#5765=EDGE_LOOP('',(#21123,#21124,#21125,#21126));
#5766=EDGE_LOOP('',(#21127));
#5767=EDGE_LOOP('',(#21128));
#5768=EDGE_LOOP('',(#21129,#21130,#21131,#21132));
#5769=EDGE_LOOP('',(#21133,#21134,#21135,#21136));
#5770=EDGE_LOOP('',(#21137));
#5771=EDGE_LOOP('',(#21138));
#5772=EDGE_LOOP('',(#21139,#21140,#21141,#21142));
#5773=EDGE_LOOP('',(#21143,#21144,#21145,#21146));
#5774=EDGE_LOOP('',(#21147));
#5775=EDGE_LOOP('',(#21148));
#5776=EDGE_LOOP('',(#21149,#21150,#21151,#21152));
#5777=EDGE_LOOP('',(#21153,#21154,#21155,#21156));
#5778=EDGE_LOOP('',(#21157));
#5779=EDGE_LOOP('',(#21158));
#5780=EDGE_LOOP('',(#21159,#21160,#21161,#21162));
#5781=EDGE_LOOP('',(#21163,#21164,#21165,#21166));
#5782=EDGE_LOOP('',(#21167));
#5783=EDGE_LOOP('',(#21168));
#5784=EDGE_LOOP('',(#21169,#21170,#21171,#21172));
#5785=EDGE_LOOP('',(#21173,#21174,#21175,#21176));
#5786=EDGE_LOOP('',(#21177));
#5787=EDGE_LOOP('',(#21178));
#5788=EDGE_LOOP('',(#21179,#21180,#21181,#21182));
#5789=EDGE_LOOP('',(#21183,#21184,#21185,#21186));
#5790=EDGE_LOOP('',(#21187));
#5791=EDGE_LOOP('',(#21188));
#5792=EDGE_LOOP('',(#21189,#21190,#21191,#21192));
#5793=EDGE_LOOP('',(#21193,#21194,#21195,#21196));
#5794=EDGE_LOOP('',(#21197));
#5795=EDGE_LOOP('',(#21198));
#5796=EDGE_LOOP('',(#21199,#21200,#21201,#21202));
#5797=EDGE_LOOP('',(#21203,#21204,#21205,#21206));
#5798=EDGE_LOOP('',(#21207));
#5799=EDGE_LOOP('',(#21208));
#5800=EDGE_LOOP('',(#21209,#21210,#21211,#21212,#21213,#21214));
#5801=EDGE_LOOP('',(#21215,#21216,#21217,#21218,#21219,#21220));
#5802=EDGE_LOOP('',(#21221,#21222,#21223,#21224));
#5803=EDGE_LOOP('',(#21225,#21226,#21227,#21228,#21229,#21230));
#5804=EDGE_LOOP('',(#21231,#21232,#21233,#21234));
#5805=EDGE_LOOP('',(#21235,#21236,#21237,#21238));
#5806=EDGE_LOOP('',(#21239));
#5807=EDGE_LOOP('',(#21240));
#5808=EDGE_LOOP('',(#21241,#21242,#21243,#21244));
#5809=EDGE_LOOP('',(#21245,#21246,#21247,#21248));
#5810=EDGE_LOOP('',(#21249));
#5811=EDGE_LOOP('',(#21250));
#5812=EDGE_LOOP('',(#21251,#21252,#21253,#21254,#21255,#21256));
#5813=EDGE_LOOP('',(#21257,#21258,#21259,#21260,#21261,#21262));
#5814=EDGE_LOOP('',(#21263,#21264,#21265,#21266));
#5815=EDGE_LOOP('',(#21267,#21268,#21269,#21270,#21271,#21272));
#5816=EDGE_LOOP('',(#21273,#21274,#21275,#21276,#21277,#21278));
#5817=EDGE_LOOP('',(#21279,#21280,#21281,#21282,#21283,#21284));
#5818=EDGE_LOOP('',(#21285,#21286,#21287,#21288));
#5819=EDGE_LOOP('',(#21289,#21290,#21291,#21292));
#5820=EDGE_LOOP('',(#21293));
#5821=EDGE_LOOP('',(#21294));
#5822=EDGE_LOOP('',(#21295,#21296,#21297,#21298));
#5823=EDGE_LOOP('',(#21299,#21300,#21301,#21302));
#5824=EDGE_LOOP('',(#21303));
#5825=EDGE_LOOP('',(#21304));
#5826=EDGE_LOOP('',(#21305,#21306,#21307,#21308));
#5827=EDGE_LOOP('',(#21309,#21310,#21311,#21312));
#5828=EDGE_LOOP('',(#21313));
#5829=EDGE_LOOP('',(#21314));
#5830=EDGE_LOOP('',(#21315));
#5831=EDGE_LOOP('',(#21316));
#5832=EDGE_LOOP('',(#21317));
#5833=EDGE_LOOP('',(#21318));
#5834=EDGE_LOOP('',(#21319));
#5835=EDGE_LOOP('',(#21320));
#5836=EDGE_LOOP('',(#21321));
#5837=EDGE_LOOP('',(#21322));
#5838=EDGE_LOOP('',(#21323));
#5839=EDGE_LOOP('',(#21324));
#5840=EDGE_LOOP('',(#21325));
#5841=EDGE_LOOP('',(#21326));
#5842=EDGE_LOOP('',(#21327));
#5843=EDGE_LOOP('',(#21328));
#5844=EDGE_LOOP('',(#21329));
#5845=EDGE_LOOP('',(#21330));
#5846=EDGE_LOOP('',(#21331));
#5847=EDGE_LOOP('',(#21332));
#5848=EDGE_LOOP('',(#21333));
#5849=EDGE_LOOP('',(#21334));
#5850=EDGE_LOOP('',(#21335));
#5851=EDGE_LOOP('',(#21336));
#5852=EDGE_LOOP('',(#21337));
#5853=EDGE_LOOP('',(#21338));
#5854=EDGE_LOOP('',(#21339));
#5855=EDGE_LOOP('',(#21340));
#5856=EDGE_LOOP('',(#21341));
#5857=EDGE_LOOP('',(#21342));
#5858=EDGE_LOOP('',(#21343));
#5859=EDGE_LOOP('',(#21344));
#5860=EDGE_LOOP('',(#21345));
#5861=EDGE_LOOP('',(#21346));
#5862=EDGE_LOOP('',(#21347));
#5863=EDGE_LOOP('',(#21348));
#5864=EDGE_LOOP('',(#21349));
#5865=EDGE_LOOP('',(#21350));
#5866=EDGE_LOOP('',(#21351));
#5867=EDGE_LOOP('',(#21352));
#5868=EDGE_LOOP('',(#21353));
#5869=EDGE_LOOP('',(#21354));
#5870=EDGE_LOOP('',(#21355,#21356,#21357,#21358));
#5871=EDGE_LOOP('',(#21359,#21360,#21361,#21362));
#5872=EDGE_LOOP('',(#21363,#21364,#21365,#21366));
#5873=EDGE_LOOP('',(#21367,#21368,#21369,#21370));
#5874=EDGE_LOOP('',(#21371,#21372,#21373,#21374));
#5875=EDGE_LOOP('',(#21375,#21376,#21377,#21378));
#5876=EDGE_LOOP('',(#21379,#21380,#21381,#21382));
#5877=EDGE_LOOP('',(#21383,#21384,#21385,#21386));
#5878=EDGE_LOOP('',(#21387,#21388,#21389,#21390));
#5879=EDGE_LOOP('',(#21391,#21392,#21393,#21394));
#5880=EDGE_LOOP('',(#21395,#21396,#21397,#21398));
#5881=EDGE_LOOP('',(#21399,#21400,#21401,#21402));
#5882=EDGE_LOOP('',(#21403,#21404,#21405,#21406));
#5883=EDGE_LOOP('',(#21407,#21408,#21409,#21410,#21411,#21412));
#5884=EDGE_LOOP('',(#21413,#21414,#21415,#21416,#21417,#21418));
#5885=EDGE_LOOP('',(#21419,#21420,#21421,#21422));
#5886=EDGE_LOOP('',(#21423,#21424,#21425,#21426));
#5887=EDGE_LOOP('',(#21427,#21428,#21429,#21430));
#5888=EDGE_LOOP('',(#21431,#21432,#21433,#21434));
#5889=EDGE_LOOP('',(#21435,#21436,#21437,#21438));
#5890=EDGE_LOOP('',(#21439,#21440,#21441,#21442));
#5891=EDGE_LOOP('',(#21443,#21444,#21445,#21446));
#5892=EDGE_LOOP('',(#21447,#21448,#21449,#21450));
#5893=EDGE_LOOP('',(#21451,#21452,#21453,#21454));
#5894=EDGE_LOOP('',(#21455,#21456,#21457,#21458));
#5895=EDGE_LOOP('',(#21459,#21460,#21461,#21462));
#5896=EDGE_LOOP('',(#21463,#21464,#21465,#21466));
#5897=EDGE_LOOP('',(#21467,#21468,#21469,#21470));
#5898=EDGE_LOOP('',(#21471,#21472,#21473,#21474));
#5899=EDGE_LOOP('',(#21475,#21476,#21477,#21478));
#5900=EDGE_LOOP('',(#21479,#21480,#21481,#21482));
#5901=EDGE_LOOP('',(#21483,#21484,#21485,#21486));
#5902=EDGE_LOOP('',(#21487,#21488,#21489,#21490));
#5903=EDGE_LOOP('',(#21491,#21492,#21493,#21494));
#5904=EDGE_LOOP('',(#21495,#21496,#21497,#21498));
#5905=EDGE_LOOP('',(#21499,#21500,#21501,#21502));
#5906=EDGE_LOOP('',(#21503,#21504,#21505,#21506));
#5907=EDGE_LOOP('',(#21507,#21508,#21509,#21510));
#5908=EDGE_LOOP('',(#21511,#21512,#21513,#21514));
#5909=EDGE_LOOP('',(#21515,#21516,#21517,#21518));
#5910=EDGE_LOOP('',(#21519,#21520,#21521,#21522));
#5911=EDGE_LOOP('',(#21523,#21524,#21525,#21526));
#5912=EDGE_LOOP('',(#21527,#21528,#21529,#21530));
#5913=EDGE_LOOP('',(#21531,#21532,#21533,#21534));
#5914=EDGE_LOOP('',(#21535,#21536,#21537,#21538));
#5915=EDGE_LOOP('',(#21539,#21540,#21541,#21542));
#5916=EDGE_LOOP('',(#21543,#21544,#21545,#21546));
#5917=EDGE_LOOP('',(#21547,#21548,#21549,#21550));
#5918=EDGE_LOOP('',(#21551,#21552,#21553,#21554));
#5919=EDGE_LOOP('',(#21555,#21556,#21557,#21558));
#5920=EDGE_LOOP('',(#21559,#21560,#21561,#21562));
#5921=EDGE_LOOP('',(#21563,#21564,#21565,#21566));
#5922=EDGE_LOOP('',(#21567,#21568,#21569,#21570));
#5923=EDGE_LOOP('',(#21571,#21572,#21573,#21574));
#5924=EDGE_LOOP('',(#21575,#21576,#21577,#21578));
#5925=EDGE_LOOP('',(#21579,#21580,#21581,#21582));
#5926=EDGE_LOOP('',(#21583,#21584,#21585,#21586));
#5927=EDGE_LOOP('',(#21587,#21588,#21589,#21590));
#5928=EDGE_LOOP('',(#21591,#21592,#21593,#21594));
#5929=EDGE_LOOP('',(#21595,#21596,#21597,#21598));
#5930=EDGE_LOOP('',(#21599,#21600,#21601,#21602));
#5931=EDGE_LOOP('',(#21603,#21604,#21605,#21606));
#5932=EDGE_LOOP('',(#21607,#21608,#21609,#21610));
#5933=EDGE_LOOP('',(#21611,#21612,#21613,#21614));
#5934=EDGE_LOOP('',(#21615,#21616,#21617,#21618));
#5935=EDGE_LOOP('',(#21619,#21620,#21621,#21622));
#5936=EDGE_LOOP('',(#21623,#21624,#21625,#21626));
#5937=EDGE_LOOP('',(#21627,#21628,#21629,#21630));
#5938=EDGE_LOOP('',(#21631,#21632,#21633,#21634));
#5939=EDGE_LOOP('',(#21635,#21636,#21637,#21638));
#5940=EDGE_LOOP('',(#21639,#21640,#21641,#21642));
#5941=EDGE_LOOP('',(#21643,#21644,#21645,#21646));
#5942=EDGE_LOOP('',(#21647,#21648,#21649,#21650,#21651,#21652));
#5943=EDGE_LOOP('',(#21653,#21654,#21655,#21656,#21657,#21658));
#5944=EDGE_LOOP('',(#21659,#21660,#21661,#21662));
#5945=EDGE_LOOP('',(#21663));
#5946=EDGE_LOOP('',(#21664));
#5947=EDGE_LOOP('',(#21665));
#5948=EDGE_LOOP('',(#21666));
#5949=EDGE_LOOP('',(#21667));
#5950=EDGE_LOOP('',(#21668));
#5951=EDGE_LOOP('',(#21669));
#5952=EDGE_LOOP('',(#21670));
#5953=EDGE_LOOP('',(#21671));
#5954=EDGE_LOOP('',(#21672));
#5955=EDGE_LOOP('',(#21673));
#5956=EDGE_LOOP('',(#21674));
#5957=EDGE_LOOP('',(#21675));
#5958=EDGE_LOOP('',(#21676));
#5959=EDGE_LOOP('',(#21677));
#5960=EDGE_LOOP('',(#21678));
#5961=EDGE_LOOP('',(#21679));
#5962=EDGE_LOOP('',(#21680));
#5963=EDGE_LOOP('',(#21681));
#5964=EDGE_LOOP('',(#21682));
#5965=EDGE_LOOP('',(#21683));
#5966=EDGE_LOOP('',(#21684));
#5967=EDGE_LOOP('',(#21685));
#5968=EDGE_LOOP('',(#21686));
#5969=EDGE_LOOP('',(#21687));
#5970=EDGE_LOOP('',(#21688));
#5971=EDGE_LOOP('',(#21689));
#5972=EDGE_LOOP('',(#21690));
#5973=EDGE_LOOP('',(#21691));
#5974=EDGE_LOOP('',(#21692));
#5975=EDGE_LOOP('',(#21693));
#5976=EDGE_LOOP('',(#21694));
#5977=EDGE_LOOP('',(#21695));
#5978=EDGE_LOOP('',(#21696));
#5979=EDGE_LOOP('',(#21697));
#5980=EDGE_LOOP('',(#21698));
#5981=EDGE_LOOP('',(#21699));
#5982=EDGE_LOOP('',(#21700));
#5983=EDGE_LOOP('',(#21701));
#5984=EDGE_LOOP('',(#21702));
#5985=EDGE_LOOP('',(#21703));
#5986=EDGE_LOOP('',(#21704));
#5987=EDGE_LOOP('',(#21705,#21706,#21707,#21708));
#5988=EDGE_LOOP('',(#21709,#21710,#21711,#21712));
#5989=EDGE_LOOP('',(#21713,#21714,#21715,#21716));
#5990=EDGE_LOOP('',(#21717,#21718,#21719,#21720));
#5991=EDGE_LOOP('',(#21721,#21722,#21723,#21724));
#5992=EDGE_LOOP('',(#21725,#21726,#21727,#21728));
#5993=EDGE_LOOP('',(#21729,#21730,#21731,#21732));
#5994=EDGE_LOOP('',(#21733,#21734,#21735,#21736));
#5995=EDGE_LOOP('',(#21737,#21738,#21739,#21740));
#5996=EDGE_LOOP('',(#21741,#21742,#21743,#21744));
#5997=EDGE_LOOP('',(#21745,#21746,#21747,#21748));
#5998=EDGE_LOOP('',(#21749,#21750,#21751,#21752));
#5999=EDGE_LOOP('',(#21753,#21754,#21755,#21756));
#6000=EDGE_LOOP('',(#21757,#21758,#21759,#21760));
#6001=EDGE_LOOP('',(#21761,#21762,#21763,#21764));
#6002=EDGE_LOOP('',(#21765,#21766,#21767,#21768));
#6003=EDGE_LOOP('',(#21769,#21770,#21771,#21772));
#6004=EDGE_LOOP('',(#21773,#21774,#21775,#21776));
#6005=EDGE_LOOP('',(#21777,#21778,#21779,#21780));
#6006=EDGE_LOOP('',(#21781,#21782,#21783,#21784));
#6007=EDGE_LOOP('',(#21785,#21786,#21787,#21788));
#6008=EDGE_LOOP('',(#21789,#21790,#21791,#21792));
#6009=EDGE_LOOP('',(#21793,#21794,#21795,#21796));
#6010=EDGE_LOOP('',(#21797,#21798,#21799,#21800));
#6011=EDGE_LOOP('',(#21801,#21802,#21803,#21804));
#6012=EDGE_LOOP('',(#21805,#21806,#21807,#21808));
#6013=EDGE_LOOP('',(#21809,#21810,#21811,#21812));
#6014=EDGE_LOOP('',(#21813,#21814,#21815,#21816));
#6015=EDGE_LOOP('',(#21817,#21818,#21819,#21820));
#6016=EDGE_LOOP('',(#21821,#21822,#21823,#21824));
#6017=EDGE_LOOP('',(#21825,#21826,#21827,#21828));
#6018=EDGE_LOOP('',(#21829,#21830,#21831,#21832));
#6019=EDGE_LOOP('',(#21833,#21834,#21835,#21836));
#6020=EDGE_LOOP('',(#21837,#21838,#21839,#21840));
#6021=EDGE_LOOP('',(#21841,#21842,#21843,#21844));
#6022=EDGE_LOOP('',(#21845,#21846,#21847,#21848));
#6023=EDGE_LOOP('',(#21849,#21850,#21851,#21852));
#6024=EDGE_LOOP('',(#21853,#21854,#21855,#21856));
#6025=EDGE_LOOP('',(#21857,#21858,#21859,#21860));
#6026=EDGE_LOOP('',(#21861,#21862,#21863,#21864));
#6027=EDGE_LOOP('',(#21865,#21866,#21867,#21868));
#6028=EDGE_LOOP('',(#21869,#21870,#21871,#21872));
#6029=EDGE_LOOP('',(#21873,#21874,#21875,#21876));
#6030=EDGE_LOOP('',(#21877,#21878,#21879,#21880));
#6031=EDGE_LOOP('',(#21881,#21882,#21883,#21884));
#6032=EDGE_LOOP('',(#21885,#21886,#21887,#21888));
#6033=EDGE_LOOP('',(#21889,#21890,#21891,#21892));
#6034=EDGE_LOOP('',(#21893,#21894,#21895,#21896));
#6035=EDGE_LOOP('',(#21897,#21898,#21899,#21900));
#6036=EDGE_LOOP('',(#21901,#21902,#21903,#21904));
#6037=EDGE_LOOP('',(#21905,#21906,#21907,#21908));
#6038=EDGE_LOOP('',(#21909,#21910,#21911,#21912));
#6039=EDGE_LOOP('',(#21913,#21914,#21915,#21916));
#6040=EDGE_LOOP('',(#21917,#21918,#21919,#21920));
#6041=EDGE_LOOP('',(#21921,#21922,#21923,#21924));
#6042=EDGE_LOOP('',(#21925,#21926,#21927,#21928));
#7913=LINE('',#43745,#10219);
#7914=LINE('',#43749,#10220);
#7915=LINE('',#43758,#10221);
#7916=LINE('',#43762,#10222);
#7917=LINE('',#43771,#10223);
#7918=LINE('',#43775,#10224);
#7919=LINE('',#43784,#10225);
#7920=LINE('',#43788,#10226);
#7921=LINE('',#43797,#10227);
#7922=LINE('',#43801,#10228);
#7923=LINE('',#43810,#10229);
#7924=LINE('',#43814,#10230);
#7925=LINE('',#43823,#10231);
#7926=LINE('',#43827,#10232);
#7927=LINE('',#43836,#10233);
#7928=LINE('',#43840,#10234);
#7929=LINE('',#43849,#10235);
#7930=LINE('',#43854,#10236);
#7931=LINE('',#43861,#10237);
#7932=LINE('',#43863,#10238);
#7933=LINE('',#43865,#10239);
#7934=LINE('',#43867,#10240);
#7935=LINE('',#43869,#10241);
#7936=LINE('',#43870,#10242);
#7937=LINE('',#43873,#10243);
#7938=LINE('',#43875,#10244);
#7939=LINE('',#43877,#10245);
#7940=LINE('',#43879,#10246);
#7941=LINE('',#43880,#10247);
#7942=LINE('',#43883,#10248);
#7943=LINE('',#43884,#10249);
#7944=LINE('',#43887,#10250);
#7945=LINE('',#43889,#10251);
#7946=LINE('',#43891,#10252);
#7947=LINE('',#43892,#10253);
#7948=LINE('',#43897,#10254);
#7949=LINE('',#43901,#10255);
#7950=LINE('',#43910,#10256);
#7951=LINE('',#43914,#10257);
#7952=LINE('',#43922,#10258);
#7953=LINE('',#43924,#10259);
#7954=LINE('',#43926,#10260);
#7955=LINE('',#43928,#10261);
#7956=LINE('',#43930,#10262);
#7957=LINE('',#43931,#10263);
#7958=LINE('',#43934,#10264);
#7959=LINE('',#43936,#10265);
#7960=LINE('',#43938,#10266);
#7961=LINE('',#43940,#10267);
#7962=LINE('',#43941,#10268);
#7963=LINE('',#43944,#10269);
#7964=LINE('',#43945,#10270);
#7965=LINE('',#43948,#10271);
#7966=LINE('',#43950,#10272);
#7967=LINE('',#43952,#10273);
#7968=LINE('',#43953,#10274);
#7969=LINE('',#43956,#10275);
#7970=LINE('',#43958,#10276);
#7971=LINE('',#43959,#10277);
#7972=LINE('',#43962,#10278);
#7973=LINE('',#43964,#10279);
#7974=LINE('',#43965,#10280);
#7975=LINE('',#43970,#10281);
#7976=LINE('',#43974,#10282);
#7977=LINE('',#43983,#10283);
#7978=LINE('',#43987,#10284);
#7979=LINE('',#43995,#10285);
#7980=LINE('',#43997,#10286);
#7981=LINE('',#43998,#10287);
#7982=LINE('',#44082,#10288);
#7983=LINE('',#44084,#10289);
#7984=LINE('',#44086,#10290);
#7985=LINE('',#44088,#10291);
#7986=LINE('',#44090,#10292);
#7987=LINE('',#44092,#10293);
#7988=LINE('',#44094,#10294);
#7989=LINE('',#44097,#10295);
#7990=LINE('',#44102,#10296);
#7991=LINE('',#44105,#10297);
#7992=LINE('',#44110,#10298);
#7993=LINE('',#44112,#10299);
#7994=LINE('',#44114,#10300);
#7995=LINE('',#44116,#10301);
#7996=LINE('',#44118,#10302);
#7997=LINE('',#44120,#10303);
#7998=LINE('',#44123,#10304);
#7999=LINE('',#44128,#10305);
#8000=LINE('',#44131,#10306);
#8001=LINE('',#44136,#10307);
#8002=LINE('',#44139,#10308);
#8003=LINE('',#44144,#10309);
#8004=LINE('',#44147,#10310);
#8005=LINE('',#44152,#10311);
#8006=LINE('',#44155,#10312);
#8007=LINE('',#44160,#10313);
#8008=LINE('',#44163,#10314);
#8009=LINE('',#44168,#10315);
#8010=LINE('',#44171,#10316);
#8011=LINE('',#44176,#10317);
#8012=LINE('',#44179,#10318);
#8013=LINE('',#44184,#10319);
#8014=LINE('',#44187,#10320);
#8015=LINE('',#44192,#10321);
#8016=LINE('',#44195,#10322);
#8017=LINE('',#44200,#10323);
#8018=LINE('',#44203,#10324);
#8019=LINE('',#44208,#10325);
#8020=LINE('',#44211,#10326);
#8021=LINE('',#44216,#10327);
#8022=LINE('',#44218,#10328);
#8023=LINE('',#44220,#10329);
#8024=LINE('',#44223,#10330);
#8025=LINE('',#44228,#10331);
#8026=LINE('',#44231,#10332);
#8027=LINE('',#44236,#10333);
#8028=LINE('',#44239,#10334);
#8029=LINE('',#44244,#10335);
#8030=LINE('',#44247,#10336);
#8031=LINE('',#44252,#10337);
#8032=LINE('',#44255,#10338);
#8033=LINE('',#44260,#10339);
#8034=LINE('',#44263,#10340);
#8035=LINE('',#44268,#10341);
#8036=LINE('',#44271,#10342);
#8037=LINE('',#44276,#10343);
#8038=LINE('',#44279,#10344);
#8039=LINE('',#44284,#10345);
#8040=LINE('',#44287,#10346);
#8041=LINE('',#44292,#10347);
#8042=LINE('',#44295,#10348);
#8043=LINE('',#44300,#10349);
#8044=LINE('',#44303,#10350);
#8045=LINE('',#44308,#10351);
#8046=LINE('',#44311,#10352);
#8047=LINE('',#44316,#10353);
#8048=LINE('',#44319,#10354);
#8049=LINE('',#44324,#10355);
#8050=LINE('',#44327,#10356);
#8051=LINE('',#44332,#10357);
#8052=LINE('',#44335,#10358);
#8053=LINE('',#44340,#10359);
#8054=LINE('',#44342,#10360);
#8055=LINE('',#44343,#10361);
#8056=LINE('',#44345,#10362);
#8057=LINE('',#44432,#10363);
#8058=LINE('',#44434,#10364);
#8059=LINE('',#44436,#10365);
#8060=LINE('',#44438,#10366);
#8061=LINE('',#44440,#10367);
#8062=LINE('',#44442,#10368);
#8063=LINE('',#44444,#10369);
#8064=LINE('',#44446,#10370);
#8065=LINE('',#44449,#10371);
#8066=LINE('',#44452,#10372);
#8067=LINE('',#44455,#10373);
#8068=LINE('',#44458,#10374);
#8069=LINE('',#44461,#10375);
#8070=LINE('',#44464,#10376);
#8071=LINE('',#44467,#10377);
#8072=LINE('',#44470,#10378);
#8073=LINE('',#44473,#10379);
#8074=LINE('',#44476,#10380);
#8075=LINE('',#44479,#10381);
#8076=LINE('',#44482,#10382);
#8077=LINE('',#44485,#10383);
#8078=LINE('',#44488,#10384);
#8079=LINE('',#44491,#10385);
#8080=LINE('',#44494,#10386);
#8081=LINE('',#44497,#10387);
#8082=LINE('',#44500,#10388);
#8083=LINE('',#44503,#10389);
#8084=LINE('',#44506,#10390);
#8085=LINE('',#44508,#10391);
#8086=LINE('',#44510,#10392);
#8087=LINE('',#44512,#10393);
#8088=LINE('',#44514,#10394);
#8089=LINE('',#44516,#10395);
#8090=LINE('',#44518,#10396);
#8091=LINE('',#44520,#10397);
#8092=LINE('',#44522,#10398);
#8093=LINE('',#44524,#10399);
#8094=LINE('',#44526,#10400);
#8095=LINE('',#44528,#10401);
#8096=LINE('',#44530,#10402);
#8097=LINE('',#44532,#10403);
#8098=LINE('',#44534,#10404);
#8099=LINE('',#44536,#10405);
#8100=LINE('',#44538,#10406);
#8101=LINE('',#44540,#10407);
#8102=LINE('',#44542,#10408);
#8103=LINE('',#44544,#10409);
#8104=LINE('',#44546,#10410);
#8105=LINE('',#44548,#10411);
#8106=LINE('',#44550,#10412);
#8107=LINE('',#44553,#10413);
#8108=LINE('',#44556,#10414);
#8109=LINE('',#44559,#10415);
#8110=LINE('',#44562,#10416);
#8111=LINE('',#44564,#10417);
#10219=VECTOR('',#34812,4.75);
#10220=VECTOR('',#34817,4.5);
#10221=VECTOR('',#34828,4.75);
#10222=VECTOR('',#34833,4.5);
#10223=VECTOR('',#34844,4.75);
#10224=VECTOR('',#34849,4.5);
#10225=VECTOR('',#34860,4.75);
#10226=VECTOR('',#34865,4.5);
#10227=VECTOR('',#34876,4.75);
#10228=VECTOR('',#34881,4.5);
#10229=VECTOR('',#34892,4.75);
#10230=VECTOR('',#34897,4.5);
#10231=VECTOR('',#34908,4.75);
#10232=VECTOR('',#34913,4.5);
#10233=VECTOR('',#34924,4.75);
#10234=VECTOR('',#34929,4.5);
#10235=VECTOR('',#34940,2.25);
#10236=VECTOR('',#34947,2.);
#10237=VECTOR('',#34954,10.);
#10238=VECTOR('',#34955,10.);
#10239=VECTOR('',#34956,10.);
#10240=VECTOR('',#34957,10.);
#10241=VECTOR('',#34958,10.);
#10242=VECTOR('',#34959,10.);
#10243=VECTOR('',#34962,10.);
#10244=VECTOR('',#34963,10.);
#10245=VECTOR('',#34964,10.);
#10246=VECTOR('',#34965,10.);
#10247=VECTOR('',#34966,10.);
#10248=VECTOR('',#34969,10.);
#10249=VECTOR('',#34970,10.);
#10250=VECTOR('',#34973,10.);
#10251=VECTOR('',#34974,10.);
#10252=VECTOR('',#34975,10.);
#10253=VECTOR('',#34976,10.);
#10254=VECTOR('',#34981,3.75);
#10255=VECTOR('',#34986,3.5);
#10256=VECTOR('',#34997,3.75);
#10257=VECTOR('',#35002,3.5);
#10258=VECTOR('',#35011,10.);
#10259=VECTOR('',#35012,10.);
#10260=VECTOR('',#35013,10.);
#10261=VECTOR('',#35014,10.);
#10262=VECTOR('',#35015,10.);
#10263=VECTOR('',#35016,10.);
#10264=VECTOR('',#35019,10.);
#10265=VECTOR('',#35020,10.);
#10266=VECTOR('',#35021,10.);
#10267=VECTOR('',#35022,10.);
#10268=VECTOR('',#35023,10.);
#10269=VECTOR('',#35026,10.);
#10270=VECTOR('',#35027,10.);
#10271=VECTOR('',#35030,10.);
#10272=VECTOR('',#35031,10.);
#10273=VECTOR('',#35032,10.);
#10274=VECTOR('',#35033,10.);
#10275=VECTOR('',#35036,10.);
#10276=VECTOR('',#35037,10.);
#10277=VECTOR('',#35038,10.);
#10278=VECTOR('',#35041,10.);
#10279=VECTOR('',#35042,10.);
#10280=VECTOR('',#35043,10.);
#10281=VECTOR('',#35048,4.75);
#10282=VECTOR('',#35053,4.5);
#10283=VECTOR('',#35064,4.75);
#10284=VECTOR('',#35069,4.5);
#10285=VECTOR('',#35080,4.75);
#10286=VECTOR('',#35083,10.);
#10287=VECTOR('',#35084,10.);
#10288=VECTOR('',#35169,4.75);
#10289=VECTOR('',#35172,4.75);
#10290=VECTOR('',#35175,4.75);
#10291=VECTOR('',#35178,4.75);
#10292=VECTOR('',#35181,4.75);
#10293=VECTOR('',#35184,4.75);
#10294=VECTOR('',#35187,4.75);
#10295=VECTOR('',#35190,7.3);
#10296=VECTOR('',#35197,7.05);
#10297=VECTOR('',#35200,7.3);
#10298=VECTOR('',#35207,7.05);
#10299=VECTOR('',#35210,4.75);
#10300=VECTOR('',#35213,4.75);
#10301=VECTOR('',#35216,10.);
#10302=VECTOR('',#35219,10.);
#10303=VECTOR('',#35222,10.);
#10304=VECTOR('',#35225,4.3);
#10305=VECTOR('',#35232,4.05);
#10306=VECTOR('',#35235,4.3);
#10307=VECTOR('',#35242,4.05);
#10308=VECTOR('',#35245,4.3);
#10309=VECTOR('',#35252,4.05);
#10310=VECTOR('',#35255,4.3);
#10311=VECTOR('',#35262,4.05);
#10312=VECTOR('',#35265,4.3);
#10313=VECTOR('',#35272,4.05);
#10314=VECTOR('',#35275,4.3);
#10315=VECTOR('',#35282,4.05);
#10316=VECTOR('',#35285,4.3);
#10317=VECTOR('',#35292,4.05);
#10318=VECTOR('',#35295,4.3);
#10319=VECTOR('',#35302,4.05);
#10320=VECTOR('',#35305,4.3);
#10321=VECTOR('',#35312,4.05);
#10322=VECTOR('',#35315,4.3);
#10323=VECTOR('',#35322,4.05);
#10324=VECTOR('',#35325,4.3);
#10325=VECTOR('',#35332,4.05);
#10326=VECTOR('',#35335,4.3);
#10327=VECTOR('',#35342,4.05);
#10328=VECTOR('',#35345,3.75);
#10329=VECTOR('',#35348,3.75);
#10330=VECTOR('',#35351,4.3);
#10331=VECTOR('',#35358,4.05);
#10332=VECTOR('',#35361,4.3);
#10333=VECTOR('',#35368,4.05);
#10334=VECTOR('',#35371,4.3);
#10335=VECTOR('',#35378,4.05);
#10336=VECTOR('',#35381,4.3);
#10337=VECTOR('',#35388,4.05);
#10338=VECTOR('',#35391,4.3);
#10339=VECTOR('',#35398,4.05);
#10340=VECTOR('',#35401,4.3);
#10341=VECTOR('',#35408,4.05);
#10342=VECTOR('',#35411,4.3);
#10343=VECTOR('',#35418,4.05);
#10344=VECTOR('',#35421,4.3);
#10345=VECTOR('',#35428,4.05);
#10346=VECTOR('',#35431,7.75);
#10347=VECTOR('',#35438,7.5);
#10348=VECTOR('',#35441,7.75);
#10349=VECTOR('',#35448,7.5);
#10350=VECTOR('',#35451,7.75);
#10351=VECTOR('',#35458,7.5);
#10352=VECTOR('',#35461,7.75);
#10353=VECTOR('',#35468,7.5);
#10354=VECTOR('',#35471,7.75);
#10355=VECTOR('',#35478,7.5);
#10356=VECTOR('',#35481,7.75);
#10357=VECTOR('',#35488,7.5);
#10358=VECTOR('',#35491,7.75);
#10359=VECTOR('',#35498,7.5);
#10360=VECTOR('',#35501,10.);
#10361=VECTOR('',#35502,10.);
#10362=VECTOR('',#35505,10.);
#10363=VECTOR('',#35594,2.25);
#10364=VECTOR('',#35597,7.75);
#10365=VECTOR('',#35600,7.75);
#10366=VECTOR('',#35603,7.75);
#10367=VECTOR('',#35606,7.75);
#10368=VECTOR('',#35609,7.75);
#10369=VECTOR('',#35612,7.75);
#10370=VECTOR('',#35615,7.75);
#10371=VECTOR('',#35618,7.25);
#10372=VECTOR('',#35623,7.);
#10373=VECTOR('',#35626,7.25);
#10374=VECTOR('',#35631,7.);
#10375=VECTOR('',#35634,7.25);
#10376=VECTOR('',#35639,7.);
#10377=VECTOR('',#35642,7.25);
#10378=VECTOR('',#35647,7.);
#10379=VECTOR('',#35650,7.25);
#10380=VECTOR('',#35655,7.);
#10381=VECTOR('',#35658,7.25);
#10382=VECTOR('',#35663,7.);
#10383=VECTOR('',#35666,7.25);
#10384=VECTOR('',#35671,7.);
#10385=VECTOR('',#35674,7.25);
#10386=VECTOR('',#35679,7.);
#10387=VECTOR('',#35682,7.25);
#10388=VECTOR('',#35687,7.);
#10389=VECTOR('',#35690,7.25);
#10390=VECTOR('',#35695,7.);
#10391=VECTOR('',#35698,4.3);
#10392=VECTOR('',#35701,4.3);
#10393=VECTOR('',#35704,4.3);
#10394=VECTOR('',#35707,4.3);
#10395=VECTOR('',#35710,4.3);
#10396=VECTOR('',#35713,4.3);
#10397=VECTOR('',#35716,4.3);
#10398=VECTOR('',#35719,4.3);
#10399=VECTOR('',#35722,4.3);
#10400=VECTOR('',#35725,4.3);
#10401=VECTOR('',#35728,4.3);
#10402=VECTOR('',#35731,4.3);
#10403=VECTOR('',#35734,4.3);
#10404=VECTOR('',#35737,4.3);
#10405=VECTOR('',#35740,4.3);
#10406=VECTOR('',#35743,4.3);
#10407=VECTOR('',#35746,4.3);
#10408=VECTOR('',#35749,4.3);
#10409=VECTOR('',#35752,4.3);
#10410=VECTOR('',#35755,4.3);
#10411=VECTOR('',#35758,7.3);
#10412=VECTOR('',#35761,7.3);
#10413=VECTOR('',#35764,6.75);
#10414=VECTOR('',#35769,6.5);
#10415=VECTOR('',#35772,6.75);
#10416=VECTOR('',#35777,6.5);
#10417=VECTOR('',#35780,4.2379);
#12578=VERTEX_POINT('',#43742);
#12579=VERTEX_POINT('',#43744);
#12580=VERTEX_POINT('',#43748);
#12581=VERTEX_POINT('',#43752);
#12582=VERTEX_POINT('',#43755);
#12583=VERTEX_POINT('',#43757);
#12584=VERTEX_POINT('',#43761);
#12585=VERTEX_POINT('',#43765);
#12586=VERTEX_POINT('',#43768);
#12587=VERTEX_POINT('',#43770);
#12588=VERTEX_POINT('',#43774);
#12589=VERTEX_POINT('',#43778);
#12590=VERTEX_POINT('',#43781);
#12591=VERTEX_POINT('',#43783);
#12592=VERTEX_POINT('',#43787);
#12593=VERTEX_POINT('',#43791);
#12594=VERTEX_POINT('',#43794);
#12595=VERTEX_POINT('',#43796);
#12596=VERTEX_POINT('',#43800);
#12597=VERTEX_POINT('',#43804);
#12598=VERTEX_POINT('',#43807);
#12599=VERTEX_POINT('',#43809);
#12600=VERTEX_POINT('',#43813);
#12601=VERTEX_POINT('',#43817);
#12602=VERTEX_POINT('',#43820);
#12603=VERTEX_POINT('',#43822);
#12604=VERTEX_POINT('',#43826);
#12605=VERTEX_POINT('',#43830);
#12606=VERTEX_POINT('',#43833);
#12607=VERTEX_POINT('',#43835);
#12608=VERTEX_POINT('',#43839);
#12609=VERTEX_POINT('',#43843);
#12610=VERTEX_POINT('',#43846);
#12611=VERTEX_POINT('',#43848);
#12612=VERTEX_POINT('',#43852);
#12613=VERTEX_POINT('',#43856);
#12614=VERTEX_POINT('',#43859);
#12615=VERTEX_POINT('',#43860);
#12616=VERTEX_POINT('',#43862);
#12617=VERTEX_POINT('',#43864);
#12618=VERTEX_POINT('',#43866);
#12619=VERTEX_POINT('',#43868);
#12620=VERTEX_POINT('',#43872);
#12621=VERTEX_POINT('',#43874);
#12622=VERTEX_POINT('',#43876);
#12623=VERTEX_POINT('',#43878);
#12624=VERTEX_POINT('',#43882);
#12625=VERTEX_POINT('',#43886);
#12626=VERTEX_POINT('',#43888);
#12627=VERTEX_POINT('',#43890);
#12628=VERTEX_POINT('',#43894);
#12629=VERTEX_POINT('',#43896);
#12630=VERTEX_POINT('',#43900);
#12631=VERTEX_POINT('',#43904);
#12632=VERTEX_POINT('',#43907);
#12633=VERTEX_POINT('',#43909);
#12634=VERTEX_POINT('',#43913);
#12635=VERTEX_POINT('',#43917);
#12636=VERTEX_POINT('',#43920);
#12637=VERTEX_POINT('',#43921);
#12638=VERTEX_POINT('',#43923);
#12639=VERTEX_POINT('',#43925);
#12640=VERTEX_POINT('',#43927);
#12641=VERTEX_POINT('',#43929);
#12642=VERTEX_POINT('',#43933);
#12643=VERTEX_POINT('',#43935);
#12644=VERTEX_POINT('',#43937);
#12645=VERTEX_POINT('',#43939);
#12646=VERTEX_POINT('',#43943);
#12647=VERTEX_POINT('',#43947);
#12648=VERTEX_POINT('',#43949);
#12649=VERTEX_POINT('',#43951);
#12650=VERTEX_POINT('',#43955);
#12651=VERTEX_POINT('',#43957);
#12652=VERTEX_POINT('',#43961);
#12653=VERTEX_POINT('',#43963);
#12654=VERTEX_POINT('',#43967);
#12655=VERTEX_POINT('',#43969);
#12656=VERTEX_POINT('',#43973);
#12657=VERTEX_POINT('',#43977);
#12658=VERTEX_POINT('',#43980);
#12659=VERTEX_POINT('',#43982);
#12660=VERTEX_POINT('',#43986);
#12661=VERTEX_POINT('',#43990);
#12662=VERTEX_POINT('',#43993);
#12663=VERTEX_POINT('',#43999);
#12664=VERTEX_POINT('',#44001);
#12665=VERTEX_POINT('',#44003);
#12666=VERTEX_POINT('',#44005);
#12667=VERTEX_POINT('',#44007);
#12668=VERTEX_POINT('',#44009);
#12669=VERTEX_POINT('',#44011);
#12670=VERTEX_POINT('',#44013);
#12671=VERTEX_POINT('',#44015);
#12672=VERTEX_POINT('',#44017);
#12673=VERTEX_POINT('',#44019);
#12674=VERTEX_POINT('',#44021);
#12675=VERTEX_POINT('',#44023);
#12676=VERTEX_POINT('',#44025);
#12677=VERTEX_POINT('',#44027);
#12678=VERTEX_POINT('',#44029);
#12679=VERTEX_POINT('',#44031);
#12680=VERTEX_POINT('',#44033);
#12681=VERTEX_POINT('',#44035);
#12682=VERTEX_POINT('',#44037);
#12683=VERTEX_POINT('',#44039);
#12684=VERTEX_POINT('',#44041);
#12685=VERTEX_POINT('',#44043);
#12686=VERTEX_POINT('',#44045);
#12687=VERTEX_POINT('',#44047);
#12688=VERTEX_POINT('',#44049);
#12689=VERTEX_POINT('',#44051);
#12690=VERTEX_POINT('',#44053);
#12691=VERTEX_POINT('',#44055);
#12692=VERTEX_POINT('',#44057);
#12693=VERTEX_POINT('',#44059);
#12694=VERTEX_POINT('',#44061);
#12695=VERTEX_POINT('',#44063);
#12696=VERTEX_POINT('',#44065);
#12697=VERTEX_POINT('',#44067);
#12698=VERTEX_POINT('',#44069);
#12699=VERTEX_POINT('',#44071);
#12700=VERTEX_POINT('',#44073);
#12701=VERTEX_POINT('',#44075);
#12702=VERTEX_POINT('',#44077);
#12703=VERTEX_POINT('',#44079);
#12704=VERTEX_POINT('',#44096);
#12705=VERTEX_POINT('',#44100);
#12706=VERTEX_POINT('',#44104);
#12707=VERTEX_POINT('',#44108);
#12708=VERTEX_POINT('',#44122);
#12709=VERTEX_POINT('',#44126);
#12710=VERTEX_POINT('',#44130);
#12711=VERTEX_POINT('',#44134);
#12712=VERTEX_POINT('',#44138);
#12713=VERTEX_POINT('',#44142);
#12714=VERTEX_POINT('',#44146);
#12715=VERTEX_POINT('',#44150);
#12716=VERTEX_POINT('',#44154);
#12717=VERTEX_POINT('',#44158);
#12718=VERTEX_POINT('',#44162);
#12719=VERTEX_POINT('',#44166);
#12720=VERTEX_POINT('',#44170);
#12721=VERTEX_POINT('',#44174);
#12722=VERTEX_POINT('',#44178);
#12723=VERTEX_POINT('',#44182);
#12724=VERTEX_POINT('',#44186);
#12725=VERTEX_POINT('',#44190);
#12726=VERTEX_POINT('',#44194);
#12727=VERTEX_POINT('',#44198);
#12728=VERTEX_POINT('',#44202);
#12729=VERTEX_POINT('',#44206);
#12730=VERTEX_POINT('',#44210);
#12731=VERTEX_POINT('',#44214);
#12732=VERTEX_POINT('',#44222);
#12733=VERTEX_POINT('',#44226);
#12734=VERTEX_POINT('',#44230);
#12735=VERTEX_POINT('',#44234);
#12736=VERTEX_POINT('',#44238);
#12737=VERTEX_POINT('',#44242);
#12738=VERTEX_POINT('',#44246);
#12739=VERTEX_POINT('',#44250);
#12740=VERTEX_POINT('',#44254);
#12741=VERTEX_POINT('',#44258);
#12742=VERTEX_POINT('',#44262);
#12743=VERTEX_POINT('',#44266);
#12744=VERTEX_POINT('',#44270);
#12745=VERTEX_POINT('',#44274);
#12746=VERTEX_POINT('',#44278);
#12747=VERTEX_POINT('',#44282);
#12748=VERTEX_POINT('',#44286);
#12749=VERTEX_POINT('',#44290);
#12750=VERTEX_POINT('',#44294);
#12751=VERTEX_POINT('',#44298);
#12752=VERTEX_POINT('',#44302);
#12753=VERTEX_POINT('',#44306);
#12754=VERTEX_POINT('',#44310);
#12755=VERTEX_POINT('',#44314);
#12756=VERTEX_POINT('',#44318);
#12757=VERTEX_POINT('',#44322);
#12758=VERTEX_POINT('',#44326);
#12759=VERTEX_POINT('',#44330);
#12760=VERTEX_POINT('',#44334);
#12761=VERTEX_POINT('',#44338);
#12762=VERTEX_POINT('',#44347);
#12763=VERTEX_POINT('',#44349);
#12764=VERTEX_POINT('',#44351);
#12765=VERTEX_POINT('',#44353);
#12766=VERTEX_POINT('',#44355);
#12767=VERTEX_POINT('',#44357);
#12768=VERTEX_POINT('',#44359);
#12769=VERTEX_POINT('',#44361);
#12770=VERTEX_POINT('',#44363);
#12771=VERTEX_POINT('',#44365);
#12772=VERTEX_POINT('',#44367);
#12773=VERTEX_POINT('',#44369);
#12774=VERTEX_POINT('',#44371);
#12775=VERTEX_POINT('',#44373);
#12776=VERTEX_POINT('',#44375);
#12777=VERTEX_POINT('',#44377);
#12778=VERTEX_POINT('',#44379);
#12779=VERTEX_POINT('',#44381);
#12780=VERTEX_POINT('',#44383);
#12781=VERTEX_POINT('',#44385);
#12782=VERTEX_POINT('',#44387);
#12783=VERTEX_POINT('',#44389);
#12784=VERTEX_POINT('',#44391);
#12785=VERTEX_POINT('',#44393);
#12786=VERTEX_POINT('',#44395);
#12787=VERTEX_POINT('',#44397);
#12788=VERTEX_POINT('',#44399);
#12789=VERTEX_POINT('',#44401);
#12790=VERTEX_POINT('',#44403);
#12791=VERTEX_POINT('',#44405);
#12792=VERTEX_POINT('',#44407);
#12793=VERTEX_POINT('',#44409);
#12794=VERTEX_POINT('',#44411);
#12795=VERTEX_POINT('',#44413);
#12796=VERTEX_POINT('',#44415);
#12797=VERTEX_POINT('',#44417);
#12798=VERTEX_POINT('',#44419);
#12799=VERTEX_POINT('',#44421);
#12800=VERTEX_POINT('',#44423);
#12801=VERTEX_POINT('',#44425);
#12802=VERTEX_POINT('',#44427);
#12803=VERTEX_POINT('',#44429);
#12804=VERTEX_POINT('',#44448);
#12805=VERTEX_POINT('',#44454);
#12806=VERTEX_POINT('',#44460);
#12807=VERTEX_POINT('',#44466);
#12808=VERTEX_POINT('',#44472);
#12809=VERTEX_POINT('',#44478);
#12810=VERTEX_POINT('',#44484);
#12811=VERTEX_POINT('',#44490);
#12812=VERTEX_POINT('',#44496);
#12813=VERTEX_POINT('',#44502);
#12814=VERTEX_POINT('',#44552);
#12815=VERTEX_POINT('',#44558);
#15781=EDGE_CURVE('',#12578,#12578,#1196,.T.);
#15782=EDGE_CURVE('',#12578,#12579,#7913,.T.);
#15783=EDGE_CURVE('',#12579,#12579,#1197,.T.);
#15784=EDGE_CURVE('',#12578,#12580,#7914,.T.);
#15785=EDGE_CURVE('',#12580,#12580,#1198,.T.);
#15786=EDGE_CURVE('',#12581,#12581,#1199,.T.);
#15787=EDGE_CURVE('',#12582,#12582,#1200,.T.);
#15788=EDGE_CURVE('',#12582,#12583,#7915,.T.);
#15789=EDGE_CURVE('',#12583,#12583,#1201,.T.);
#15790=EDGE_CURVE('',#12582,#12584,#7916,.T.);
#15791=EDGE_CURVE('',#12584,#12584,#1202,.T.);
#15792=EDGE_CURVE('',#12585,#12585,#1203,.T.);
#15793=EDGE_CURVE('',#12586,#12586,#1204,.T.);
#15794=EDGE_CURVE('',#12586,#12587,#7917,.T.);
#15795=EDGE_CURVE('',#12587,#12587,#1205,.T.);
#15796=EDGE_CURVE('',#12586,#12588,#7918,.T.);
#15797=EDGE_CURVE('',#12588,#12588,#1206,.T.);
#15798=EDGE_CURVE('',#12589,#12589,#1207,.T.);
#15799=EDGE_CURVE('',#12590,#12590,#1208,.T.);
#15800=EDGE_CURVE('',#12590,#12591,#7919,.T.);
#15801=EDGE_CURVE('',#12591,#12591,#1209,.T.);
#15802=EDGE_CURVE('',#12590,#12592,#7920,.T.);
#15803=EDGE_CURVE('',#12592,#12592,#1210,.T.);
#15804=EDGE_CURVE('',#12593,#12593,#1211,.T.);
#15805=EDGE_CURVE('',#12594,#12594,#1212,.T.);
#15806=EDGE_CURVE('',#12594,#12595,#7921,.T.);
#15807=EDGE_CURVE('',#12595,#12595,#1213,.T.);
#15808=EDGE_CURVE('',#12594,#12596,#7922,.T.);
#15809=EDGE_CURVE('',#12596,#12596,#1214,.T.);
#15810=EDGE_CURVE('',#12597,#12597,#1215,.T.);
#15811=EDGE_CURVE('',#12598,#12598,#1216,.T.);
#15812=EDGE_CURVE('',#12598,#12599,#7923,.T.);
#15813=EDGE_CURVE('',#12599,#12599,#1217,.T.);
#15814=EDGE_CURVE('',#12598,#12600,#7924,.T.);
#15815=EDGE_CURVE('',#12600,#12600,#1218,.T.);
#15816=EDGE_CURVE('',#12601,#12601,#1219,.T.);
#15817=EDGE_CURVE('',#12602,#12602,#1220,.T.);
#15818=EDGE_CURVE('',#12602,#12603,#7925,.T.);
#15819=EDGE_CURVE('',#12603,#12603,#1221,.T.);
#15820=EDGE_CURVE('',#12602,#12604,#7926,.T.);
#15821=EDGE_CURVE('',#12604,#12604,#1222,.T.);
#15822=EDGE_CURVE('',#12605,#12605,#1223,.T.);
#15823=EDGE_CURVE('',#12606,#12606,#1224,.T.);
#15824=EDGE_CURVE('',#12606,#12607,#7927,.T.);
#15825=EDGE_CURVE('',#12607,#12607,#1225,.T.);
#15826=EDGE_CURVE('',#12606,#12608,#7928,.T.);
#15827=EDGE_CURVE('',#12608,#12608,#1226,.T.);
#15828=EDGE_CURVE('',#12609,#12609,#1227,.T.);
#15829=EDGE_CURVE('',#12610,#12610,#1228,.T.);
#15830=EDGE_CURVE('',#12610,#12611,#7929,.T.);
#15831=EDGE_CURVE('',#12611,#12611,#1229,.T.);
#15832=EDGE_CURVE('',#12612,#12612,#1230,.T.);
#15833=EDGE_CURVE('',#12612,#12610,#7930,.T.);
#15834=EDGE_CURVE('',#12613,#12613,#1231,.T.);
#15835=EDGE_CURVE('',#12614,#12615,#7931,.T.);
#15836=EDGE_CURVE('',#12615,#12616,#7932,.T.);
#15837=EDGE_CURVE('',#12616,#12617,#7933,.T.);
#15838=EDGE_CURVE('',#12617,#12618,#7934,.T.);
#15839=EDGE_CURVE('',#12618,#12619,#7935,.T.);
#15840=EDGE_CURVE('',#12619,#12614,#7936,.T.);
#15841=EDGE_CURVE('',#12619,#12620,#7937,.T.);
#15842=EDGE_CURVE('',#12621,#12620,#7938,.T.);
#15843=EDGE_CURVE('',#12622,#12621,#7939,.T.);
#15844=EDGE_CURVE('',#12622,#12623,#7940,.T.);
#15845=EDGE_CURVE('',#12623,#12614,#7941,.T.);
#15846=EDGE_CURVE('',#12624,#12618,#7942,.T.);
#15847=EDGE_CURVE('',#12620,#12624,#7943,.T.);
#15848=EDGE_CURVE('',#12625,#12617,#7944,.T.);
#15849=EDGE_CURVE('',#12625,#12626,#7945,.T.);
#15850=EDGE_CURVE('',#12626,#12627,#7946,.T.);
#15851=EDGE_CURVE('',#12624,#12627,#7947,.T.);
#15852=EDGE_CURVE('',#12628,#12628,#1232,.T.);
#15853=EDGE_CURVE('',#12628,#12629,#7948,.T.);
#15854=EDGE_CURVE('',#12629,#12629,#1233,.T.);
#15855=EDGE_CURVE('',#12628,#12630,#7949,.T.);
#15856=EDGE_CURVE('',#12630,#12630,#1234,.T.);
#15857=EDGE_CURVE('',#12631,#12631,#1235,.T.);
#15858=EDGE_CURVE('',#12632,#12632,#1236,.T.);
#15859=EDGE_CURVE('',#12632,#12633,#7950,.T.);
#15860=EDGE_CURVE('',#12633,#12633,#1237,.T.);
#15861=EDGE_CURVE('',#12632,#12634,#7951,.T.);
#15862=EDGE_CURVE('',#12634,#12634,#1238,.T.);
#15863=EDGE_CURVE('',#12635,#12635,#1239,.T.);
#15864=EDGE_CURVE('',#12636,#12637,#7952,.T.);
#15865=EDGE_CURVE('',#12637,#12638,#7953,.T.);
#15866=EDGE_CURVE('',#12638,#12639,#7954,.T.);
#15867=EDGE_CURVE('',#12639,#12640,#7955,.T.);
#15868=EDGE_CURVE('',#12640,#12641,#7956,.T.);
#15869=EDGE_CURVE('',#12641,#12636,#7957,.T.);
#15870=EDGE_CURVE('',#12638,#12642,#7958,.T.);
#15871=EDGE_CURVE('',#12643,#12642,#7959,.T.);
#15872=EDGE_CURVE('',#12643,#12644,#7960,.T.);
#15873=EDGE_CURVE('',#12644,#12645,#7961,.T.);
#15874=EDGE_CURVE('',#12645,#12639,#7962,.T.);
#15875=EDGE_CURVE('',#12646,#12637,#7963,.T.);
#15876=EDGE_CURVE('',#12642,#12646,#7964,.T.);
#15877=EDGE_CURVE('',#12647,#12636,#7965,.T.);
#15878=EDGE_CURVE('',#12647,#12648,#7966,.T.);
#15879=EDGE_CURVE('',#12648,#12649,#7967,.T.);
#15880=EDGE_CURVE('',#12646,#12649,#7968,.T.);
#15881=EDGE_CURVE('',#12627,#12650,#7969,.T.);
#15882=EDGE_CURVE('',#12650,#12651,#7970,.T.);
#15883=EDGE_CURVE('',#12651,#12621,#7971,.T.);
#15884=EDGE_CURVE('',#12649,#12652,#7972,.T.);
#15885=EDGE_CURVE('',#12652,#12653,#7973,.T.);
#15886=EDGE_CURVE('',#12653,#12643,#7974,.T.);
#15887=EDGE_CURVE('',#12654,#12654,#1240,.T.);
#15888=EDGE_CURVE('',#12654,#12655,#7975,.T.);
#15889=EDGE_CURVE('',#12655,#12655,#1241,.T.);
#15890=EDGE_CURVE('',#12654,#12656,#7976,.T.);
#15891=EDGE_CURVE('',#12656,#12656,#1242,.T.);
#15892=EDGE_CURVE('',#12657,#12657,#1243,.T.);
#15893=EDGE_CURVE('',#12658,#12658,#1244,.T.);
#15894=EDGE_CURVE('',#12658,#12659,#7977,.T.);
#15895=EDGE_CURVE('',#12659,#12659,#1245,.T.);
#15896=EDGE_CURVE('',#12658,#12660,#7978,.T.);
#15897=EDGE_CURVE('',#12660,#12660,#1246,.T.);
#15898=EDGE_CURVE('',#12661,#12661,#1247,.T.);
#15899=EDGE_CURVE('',#12662,#12662,#1248,.T.);
#15900=EDGE_CURVE('',#12662,#12604,#7979,.T.);
#15901=EDGE_CURVE('',#12626,#12644,#7980,.T.);
#15902=EDGE_CURVE('',#12645,#12625,#7981,.T.);
#15903=EDGE_CURVE('',#12663,#12663,#1249,.T.);
#15904=EDGE_CURVE('',#12664,#12664,#1250,.T.);
#15905=EDGE_CURVE('',#12665,#12665,#1251,.T.);
#15906=EDGE_CURVE('',#12666,#12666,#1252,.T.);
#15907=EDGE_CURVE('',#12667,#12667,#1253,.T.);
#15908=EDGE_CURVE('',#12668,#12668,#1254,.T.);
#15909=EDGE_CURVE('',#12669,#12669,#1255,.T.);
#15910=EDGE_CURVE('',#12670,#12670,#1256,.T.);
#15911=EDGE_CURVE('',#12671,#12671,#1257,.T.);
#15912=EDGE_CURVE('',#12672,#12672,#1258,.T.);
#15913=EDGE_CURVE('',#12673,#12673,#1259,.T.);
#15914=EDGE_CURVE('',#12674,#12674,#1260,.T.);
#15915=EDGE_CURVE('',#12675,#12675,#1261,.T.);
#15916=EDGE_CURVE('',#12676,#12676,#1262,.T.);
#15917=EDGE_CURVE('',#12677,#12677,#1263,.T.);
#15918=EDGE_CURVE('',#12678,#12678,#1264,.T.);
#15919=EDGE_CURVE('',#12679,#12679,#1265,.T.);
#15920=EDGE_CURVE('',#12680,#12680,#1266,.T.);
#15921=EDGE_CURVE('',#12681,#12681,#1267,.T.);
#15922=EDGE_CURVE('',#12682,#12682,#1268,.T.);
#15923=EDGE_CURVE('',#12683,#12683,#1269,.T.);
#15924=EDGE_CURVE('',#12684,#12684,#1270,.T.);
#15925=EDGE_CURVE('',#12685,#12685,#1271,.T.);
#15926=EDGE_CURVE('',#12686,#12686,#1272,.T.);
#15927=EDGE_CURVE('',#12687,#12687,#1273,.T.);
#15928=EDGE_CURVE('',#12688,#12688,#1274,.T.);
#15929=EDGE_CURVE('',#12689,#12689,#1275,.T.);
#15930=EDGE_CURVE('',#12690,#12690,#1276,.T.);
#15931=EDGE_CURVE('',#12691,#12691,#1277,.T.);
#15932=EDGE_CURVE('',#12692,#12692,#1278,.T.);
#15933=EDGE_CURVE('',#12693,#12693,#1279,.T.);
#15934=EDGE_CURVE('',#12694,#12694,#1280,.T.);
#15935=EDGE_CURVE('',#12695,#12695,#1281,.T.);
#15936=EDGE_CURVE('',#12696,#12696,#1282,.T.);
#15937=EDGE_CURVE('',#12697,#12697,#1283,.T.);
#15938=EDGE_CURVE('',#12698,#12698,#1284,.T.);
#15939=EDGE_CURVE('',#12699,#12699,#1285,.T.);
#15940=EDGE_CURVE('',#12700,#12700,#1286,.T.);
#15941=EDGE_CURVE('',#12701,#12701,#1287,.T.);
#15942=EDGE_CURVE('',#12702,#12702,#1288,.T.);
#15943=EDGE_CURVE('',#12703,#12703,#1289,.T.);
#15944=EDGE_CURVE('',#12663,#12600,#7982,.T.);
#15945=EDGE_CURVE('',#12703,#12596,#7983,.T.);
#15946=EDGE_CURVE('',#12664,#12592,#7984,.T.);
#15947=EDGE_CURVE('',#12702,#12588,#7985,.T.);
#15948=EDGE_CURVE('',#12665,#12584,#7986,.T.);
#15949=EDGE_CURVE('',#12701,#12580,#7987,.T.);
#15950=EDGE_CURVE('',#12666,#12608,#7988,.T.);
#15951=EDGE_CURVE('',#12700,#12704,#7989,.T.);
#15952=EDGE_CURVE('',#12704,#12704,#1290,.T.);
#15953=EDGE_CURVE('',#12705,#12705,#1291,.T.);
#15954=EDGE_CURVE('',#12705,#12704,#7990,.T.);
#15955=EDGE_CURVE('',#12667,#12706,#7991,.T.);
#15956=EDGE_CURVE('',#12706,#12706,#1292,.T.);
#15957=EDGE_CURVE('',#12707,#12707,#1293,.T.);
#15958=EDGE_CURVE('',#12707,#12706,#7992,.T.);
#15959=EDGE_CURVE('',#12699,#12660,#7993,.T.);
#15960=EDGE_CURVE('',#12668,#12656,#7994,.T.);
#15961=EDGE_CURVE('',#12653,#12650,#7995,.T.);
#15962=EDGE_CURVE('',#12616,#12640,#7996,.T.);
#15963=EDGE_CURVE('',#12651,#12652,#7997,.T.);
#15964=EDGE_CURVE('',#12669,#12708,#7998,.T.);
#15965=EDGE_CURVE('',#12708,#12708,#1294,.T.);
#15966=EDGE_CURVE('',#12709,#12709,#1295,.T.);
#15967=EDGE_CURVE('',#12709,#12708,#7999,.T.);
#15968=EDGE_CURVE('',#12698,#12710,#8000,.T.);
#15969=EDGE_CURVE('',#12710,#12710,#1296,.T.);
#15970=EDGE_CURVE('',#12711,#12711,#1297,.T.);
#15971=EDGE_CURVE('',#12711,#12710,#8001,.T.);
#15972=EDGE_CURVE('',#12670,#12712,#8002,.T.);
#15973=EDGE_CURVE('',#12712,#12712,#1298,.T.);
#15974=EDGE_CURVE('',#12713,#12713,#1299,.T.);
#15975=EDGE_CURVE('',#12713,#12712,#8003,.T.);
#15976=EDGE_CURVE('',#12697,#12714,#8004,.T.);
#15977=EDGE_CURVE('',#12714,#12714,#1300,.T.);
#15978=EDGE_CURVE('',#12715,#12715,#1301,.T.);
#15979=EDGE_CURVE('',#12715,#12714,#8005,.T.);
#15980=EDGE_CURVE('',#12671,#12716,#8006,.T.);
#15981=EDGE_CURVE('',#12716,#12716,#1302,.T.);
#15982=EDGE_CURVE('',#12717,#12717,#1303,.T.);
#15983=EDGE_CURVE('',#12717,#12716,#8007,.T.);
#15984=EDGE_CURVE('',#12696,#12718,#8008,.T.);
#15985=EDGE_CURVE('',#12718,#12718,#1304,.T.);
#15986=EDGE_CURVE('',#12719,#12719,#1305,.T.);
#15987=EDGE_CURVE('',#12719,#12718,#8009,.T.);
#15988=EDGE_CURVE('',#12672,#12720,#8010,.T.);
#15989=EDGE_CURVE('',#12720,#12720,#1306,.T.);
#15990=EDGE_CURVE('',#12721,#12721,#1307,.T.);
#15991=EDGE_CURVE('',#12721,#12720,#8011,.T.);
#15992=EDGE_CURVE('',#12695,#12722,#8012,.T.);
#15993=EDGE_CURVE('',#12722,#12722,#1308,.T.);
#15994=EDGE_CURVE('',#12723,#12723,#1309,.T.);
#15995=EDGE_CURVE('',#12723,#12722,#8013,.T.);
#15996=EDGE_CURVE('',#12673,#12724,#8014,.T.);
#15997=EDGE_CURVE('',#12724,#12724,#1310,.T.);
#15998=EDGE_CURVE('',#12725,#12725,#1311,.T.);
#15999=EDGE_CURVE('',#12725,#12724,#8015,.T.);
#16000=EDGE_CURVE('',#12694,#12726,#8016,.T.);
#16001=EDGE_CURVE('',#12726,#12726,#1312,.T.);
#16002=EDGE_CURVE('',#12727,#12727,#1313,.T.);
#16003=EDGE_CURVE('',#12727,#12726,#8017,.T.);
#16004=EDGE_CURVE('',#12674,#12728,#8018,.T.);
#16005=EDGE_CURVE('',#12728,#12728,#1314,.T.);
#16006=EDGE_CURVE('',#12729,#12729,#1315,.T.);
#16007=EDGE_CURVE('',#12729,#12728,#8019,.T.);
#16008=EDGE_CURVE('',#12693,#12730,#8020,.T.);
#16009=EDGE_CURVE('',#12730,#12730,#1316,.T.);
#16010=EDGE_CURVE('',#12731,#12731,#1317,.T.);
#16011=EDGE_CURVE('',#12731,#12730,#8021,.T.);
#16012=EDGE_CURVE('',#12675,#12634,#8022,.T.);
#16013=EDGE_CURVE('',#12692,#12630,#8023,.T.);
#16014=EDGE_CURVE('',#12676,#12732,#8024,.T.);
#16015=EDGE_CURVE('',#12732,#12732,#1318,.T.);
#16016=EDGE_CURVE('',#12733,#12733,#1319,.T.);
#16017=EDGE_CURVE('',#12733,#12732,#8025,.T.);
#16018=EDGE_CURVE('',#12691,#12734,#8026,.T.);
#16019=EDGE_CURVE('',#12734,#12734,#1320,.T.);
#16020=EDGE_CURVE('',#12735,#12735,#1321,.T.);
#16021=EDGE_CURVE('',#12735,#12734,#8027,.T.);
#16022=EDGE_CURVE('',#12677,#12736,#8028,.T.);
#16023=EDGE_CURVE('',#12736,#12736,#1322,.T.);
#16024=EDGE_CURVE('',#12737,#12737,#1323,.T.);
#16025=EDGE_CURVE('',#12737,#12736,#8029,.T.);
#16026=EDGE_CURVE('',#12690,#12738,#8030,.T.);
#16027=EDGE_CURVE('',#12738,#12738,#1324,.T.);
#16028=EDGE_CURVE('',#12739,#12739,#1325,.T.);
#16029=EDGE_CURVE('',#12739,#12738,#8031,.T.);
#16030=EDGE_CURVE('',#12678,#12740,#8032,.T.);
#16031=EDGE_CURVE('',#12740,#12740,#1326,.T.);
#16032=EDGE_CURVE('',#12741,#12741,#1327,.T.);
#16033=EDGE_CURVE('',#12741,#12740,#8033,.T.);
#16034=EDGE_CURVE('',#12689,#12742,#8034,.T.);
#16035=EDGE_CURVE('',#12742,#12742,#1328,.T.);
#16036=EDGE_CURVE('',#12743,#12743,#1329,.T.);
#16037=EDGE_CURVE('',#12743,#12742,#8035,.T.);
#16038=EDGE_CURVE('',#12679,#12744,#8036,.T.);
#16039=EDGE_CURVE('',#12744,#12744,#1330,.T.);
#16040=EDGE_CURVE('',#12745,#12745,#1331,.T.);
#16041=EDGE_CURVE('',#12745,#12744,#8037,.T.);
#16042=EDGE_CURVE('',#12688,#12746,#8038,.T.);
#16043=EDGE_CURVE('',#12746,#12746,#1332,.T.);
#16044=EDGE_CURVE('',#12747,#12747,#1333,.T.);
#16045=EDGE_CURVE('',#12747,#12746,#8039,.T.);
#16046=EDGE_CURVE('',#12680,#12748,#8040,.T.);
#16047=EDGE_CURVE('',#12748,#12748,#1334,.T.);
#16048=EDGE_CURVE('',#12749,#12749,#1335,.T.);
#16049=EDGE_CURVE('',#12749,#12748,#8041,.T.);
#16050=EDGE_CURVE('',#12687,#12750,#8042,.T.);
#16051=EDGE_CURVE('',#12750,#12750,#1336,.T.);
#16052=EDGE_CURVE('',#12751,#12751,#1337,.T.);
#16053=EDGE_CURVE('',#12751,#12750,#8043,.T.);
#16054=EDGE_CURVE('',#12681,#12752,#8044,.T.);
#16055=EDGE_CURVE('',#12752,#12752,#1338,.T.);
#16056=EDGE_CURVE('',#12753,#12753,#1339,.T.);
#16057=EDGE_CURVE('',#12753,#12752,#8045,.T.);
#16058=EDGE_CURVE('',#12686,#12754,#8046,.T.);
#16059=EDGE_CURVE('',#12754,#12754,#1340,.T.);
#16060=EDGE_CURVE('',#12755,#12755,#1341,.T.);
#16061=EDGE_CURVE('',#12755,#12754,#8047,.T.);
#16062=EDGE_CURVE('',#12682,#12756,#8048,.T.);
#16063=EDGE_CURVE('',#12756,#12756,#1342,.T.);
#16064=EDGE_CURVE('',#12757,#12757,#1343,.T.);
#16065=EDGE_CURVE('',#12757,#12756,#8049,.T.);
#16066=EDGE_CURVE('',#12685,#12758,#8050,.T.);
#16067=EDGE_CURVE('',#12758,#12758,#1344,.T.);
#16068=EDGE_CURVE('',#12759,#12759,#1345,.T.);
#16069=EDGE_CURVE('',#12759,#12758,#8051,.T.);
#16070=EDGE_CURVE('',#12683,#12760,#8052,.T.);
#16071=EDGE_CURVE('',#12760,#12760,#1346,.T.);
#16072=EDGE_CURVE('',#12761,#12761,#1347,.T.);
#16073=EDGE_CURVE('',#12761,#12760,#8053,.T.);
#16074=EDGE_CURVE('',#12623,#12647,#8054,.T.);
#16075=EDGE_CURVE('',#12641,#12615,#8055,.T.);
#16076=EDGE_CURVE('',#12648,#12622,#8056,.T.);
#16077=EDGE_CURVE('',#12762,#12762,#1348,.T.);
#16078=EDGE_CURVE('',#12763,#12763,#1349,.T.);
#16079=EDGE_CURVE('',#12764,#12764,#1350,.T.);
#16080=EDGE_CURVE('',#12765,#12765,#1351,.T.);
#16081=EDGE_CURVE('',#12766,#12766,#1352,.T.);
#16082=EDGE_CURVE('',#12767,#12767,#1353,.T.);
#16083=EDGE_CURVE('',#12768,#12768,#1354,.T.);
#16084=EDGE_CURVE('',#12769,#12769,#1355,.T.);
#16085=EDGE_CURVE('',#12770,#12770,#1356,.T.);
#16086=EDGE_CURVE('',#12771,#12771,#1357,.T.);
#16087=EDGE_CURVE('',#12772,#12772,#1358,.T.);
#16088=EDGE_CURVE('',#12773,#12773,#1359,.T.);
#16089=EDGE_CURVE('',#12774,#12774,#1360,.T.);
#16090=EDGE_CURVE('',#12775,#12775,#1361,.T.);
#16091=EDGE_CURVE('',#12776,#12776,#1362,.T.);
#16092=EDGE_CURVE('',#12777,#12777,#1363,.T.);
#16093=EDGE_CURVE('',#12778,#12778,#1364,.T.);
#16094=EDGE_CURVE('',#12779,#12779,#1365,.T.);
#16095=EDGE_CURVE('',#12780,#12780,#1366,.T.);
#16096=EDGE_CURVE('',#12781,#12781,#1367,.T.);
#16097=EDGE_CURVE('',#12782,#12782,#1368,.T.);
#16098=EDGE_CURVE('',#12783,#12783,#1369,.T.);
#16099=EDGE_CURVE('',#12784,#12784,#1370,.T.);
#16100=EDGE_CURVE('',#12785,#12785,#1371,.T.);
#16101=EDGE_CURVE('',#12786,#12786,#1372,.T.);
#16102=EDGE_CURVE('',#12787,#12787,#1373,.T.);
#16103=EDGE_CURVE('',#12788,#12788,#1374,.T.);
#16104=EDGE_CURVE('',#12789,#12789,#1375,.T.);
#16105=EDGE_CURVE('',#12790,#12790,#1376,.T.);
#16106=EDGE_CURVE('',#12791,#12791,#1377,.T.);
#16107=EDGE_CURVE('',#12792,#12792,#1378,.T.);
#16108=EDGE_CURVE('',#12793,#12793,#1379,.T.);
#16109=EDGE_CURVE('',#12794,#12794,#1380,.T.);
#16110=EDGE_CURVE('',#12795,#12795,#1381,.T.);
#16111=EDGE_CURVE('',#12796,#12796,#1382,.T.);
#16112=EDGE_CURVE('',#12797,#12797,#1383,.T.);
#16113=EDGE_CURVE('',#12798,#12798,#1384,.T.);
#16114=EDGE_CURVE('',#12799,#12799,#1385,.T.);
#16115=EDGE_CURVE('',#12800,#12800,#1386,.T.);
#16116=EDGE_CURVE('',#12801,#12801,#1387,.T.);
#16117=EDGE_CURVE('',#12802,#12802,#1388,.T.);
#16118=EDGE_CURVE('',#12803,#12803,#1389,.T.);
#16119=EDGE_CURVE('',#12762,#12612,#8057,.T.);
#16120=EDGE_CURVE('',#12803,#12761,#8058,.T.);
#16121=EDGE_CURVE('',#12763,#12759,#8059,.T.);
#16122=EDGE_CURVE('',#12802,#12757,#8060,.T.);
#16123=EDGE_CURVE('',#12764,#12755,#8061,.T.);
#16124=EDGE_CURVE('',#12801,#12753,#8062,.T.);
#16125=EDGE_CURVE('',#12765,#12751,#8063,.T.);
#16126=EDGE_CURVE('',#12800,#12749,#8064,.T.);
#16127=EDGE_CURVE('',#12766,#12804,#8065,.T.);
#16128=EDGE_CURVE('',#12804,#12804,#1390,.T.);
#16129=EDGE_CURVE('',#12804,#12657,#8066,.T.);
#16130=EDGE_CURVE('',#12799,#12805,#8067,.T.);
#16131=EDGE_CURVE('',#12805,#12805,#1391,.T.);
#16132=EDGE_CURVE('',#12805,#12661,#8068,.T.);
#16133=EDGE_CURVE('',#12767,#12806,#8069,.T.);
#16134=EDGE_CURVE('',#12806,#12806,#1392,.T.);
#16135=EDGE_CURVE('',#12806,#12605,#8070,.T.);
#16136=EDGE_CURVE('',#12798,#12807,#8071,.T.);
#16137=EDGE_CURVE('',#12807,#12807,#1393,.T.);
#16138=EDGE_CURVE('',#12807,#12601,#8072,.T.);
#16139=EDGE_CURVE('',#12768,#12808,#8073,.T.);
#16140=EDGE_CURVE('',#12808,#12808,#1394,.T.);
#16141=EDGE_CURVE('',#12808,#12597,#8074,.T.);
#16142=EDGE_CURVE('',#12797,#12809,#8075,.T.);
#16143=EDGE_CURVE('',#12809,#12809,#1395,.T.);
#16144=EDGE_CURVE('',#12809,#12593,#8076,.T.);
#16145=EDGE_CURVE('',#12769,#12810,#8077,.T.);
#16146=EDGE_CURVE('',#12810,#12810,#1396,.T.);
#16147=EDGE_CURVE('',#12810,#12589,#8078,.T.);
#16148=EDGE_CURVE('',#12796,#12811,#8079,.T.);
#16149=EDGE_CURVE('',#12811,#12811,#1397,.T.);
#16150=EDGE_CURVE('',#12811,#12585,#8080,.T.);
#16151=EDGE_CURVE('',#12770,#12812,#8081,.T.);
#16152=EDGE_CURVE('',#12812,#12812,#1398,.T.);
#16153=EDGE_CURVE('',#12812,#12581,#8082,.T.);
#16154=EDGE_CURVE('',#12795,#12813,#8083,.T.);
#16155=EDGE_CURVE('',#12813,#12813,#1399,.T.);
#16156=EDGE_CURVE('',#12813,#12609,#8084,.T.);
#16157=EDGE_CURVE('',#12771,#12747,#8085,.T.);
#16158=EDGE_CURVE('',#12794,#12745,#8086,.T.);
#16159=EDGE_CURVE('',#12772,#12743,#8087,.T.);
#16160=EDGE_CURVE('',#12793,#12741,#8088,.T.);
#16161=EDGE_CURVE('',#12773,#12739,#8089,.T.);
#16162=EDGE_CURVE('',#12792,#12737,#8090,.T.);
#16163=EDGE_CURVE('',#12774,#12735,#8091,.T.);
#16164=EDGE_CURVE('',#12791,#12733,#8092,.T.);
#16165=EDGE_CURVE('',#12775,#12709,#8093,.T.);
#16166=EDGE_CURVE('',#12790,#12711,#8094,.T.);
#16167=EDGE_CURVE('',#12776,#12713,#8095,.T.);
#16168=EDGE_CURVE('',#12789,#12715,#8096,.T.);
#16169=EDGE_CURVE('',#12777,#12717,#8097,.T.);
#16170=EDGE_CURVE('',#12788,#12719,#8098,.T.);
#16171=EDGE_CURVE('',#12778,#12721,#8099,.T.);
#16172=EDGE_CURVE('',#12787,#12723,#8100,.T.);
#16173=EDGE_CURVE('',#12779,#12725,#8101,.T.);
#16174=EDGE_CURVE('',#12786,#12727,#8102,.T.);
#16175=EDGE_CURVE('',#12780,#12729,#8103,.T.);
#16176=EDGE_CURVE('',#12785,#12731,#8104,.T.);
#16177=EDGE_CURVE('',#12781,#12705,#8105,.T.);
#16178=EDGE_CURVE('',#12784,#12707,#8106,.T.);
#16179=EDGE_CURVE('',#12782,#12814,#8107,.T.);
#16180=EDGE_CURVE('',#12814,#12814,#1400,.T.);
#16181=EDGE_CURVE('',#12814,#12635,#8108,.T.);
#16182=EDGE_CURVE('',#12783,#12815,#8109,.T.);
#16183=EDGE_CURVE('',#12815,#12815,#1401,.T.);
#16184=EDGE_CURVE('',#12815,#12631,#8110,.T.);
#16185=EDGE_CURVE('',#12684,#12613,#8111,.T.);
#21119=ORIENTED_EDGE('',*,*,#15781,.T.);
#21120=ORIENTED_EDGE('',*,*,#15782,.T.);
#21121=ORIENTED_EDGE('',*,*,#15783,.T.);
#21122=ORIENTED_EDGE('',*,*,#15782,.F.);
#21123=ORIENTED_EDGE('',*,*,#15781,.F.);
#21124=ORIENTED_EDGE('',*,*,#15784,.T.);
#21125=ORIENTED_EDGE('',*,*,#15785,.F.);
#21126=ORIENTED_EDGE('',*,*,#15784,.F.);
#21127=ORIENTED_EDGE('',*,*,#15786,.F.);
#21128=ORIENTED_EDGE('',*,*,#15783,.F.);
#21129=ORIENTED_EDGE('',*,*,#15787,.T.);
#21130=ORIENTED_EDGE('',*,*,#15788,.T.);
#21131=ORIENTED_EDGE('',*,*,#15789,.T.);
#21132=ORIENTED_EDGE('',*,*,#15788,.F.);
#21133=ORIENTED_EDGE('',*,*,#15787,.F.);
#21134=ORIENTED_EDGE('',*,*,#15790,.T.);
#21135=ORIENTED_EDGE('',*,*,#15791,.F.);
#21136=ORIENTED_EDGE('',*,*,#15790,.F.);
#21137=ORIENTED_EDGE('',*,*,#15792,.F.);
#21138=ORIENTED_EDGE('',*,*,#15789,.F.);
#21139=ORIENTED_EDGE('',*,*,#15793,.T.);
#21140=ORIENTED_EDGE('',*,*,#15794,.T.);
#21141=ORIENTED_EDGE('',*,*,#15795,.T.);
#21142=ORIENTED_EDGE('',*,*,#15794,.F.);
#21143=ORIENTED_EDGE('',*,*,#15793,.F.);
#21144=ORIENTED_EDGE('',*,*,#15796,.T.);
#21145=ORIENTED_EDGE('',*,*,#15797,.F.);
#21146=ORIENTED_EDGE('',*,*,#15796,.F.);
#21147=ORIENTED_EDGE('',*,*,#15798,.F.);
#21148=ORIENTED_EDGE('',*,*,#15795,.F.);
#21149=ORIENTED_EDGE('',*,*,#15799,.T.);
#21150=ORIENTED_EDGE('',*,*,#15800,.T.);
#21151=ORIENTED_EDGE('',*,*,#15801,.T.);
#21152=ORIENTED_EDGE('',*,*,#15800,.F.);
#21153=ORIENTED_EDGE('',*,*,#15799,.F.);
#21154=ORIENTED_EDGE('',*,*,#15802,.T.);
#21155=ORIENTED_EDGE('',*,*,#15803,.F.);
#21156=ORIENTED_EDGE('',*,*,#15802,.F.);
#21157=ORIENTED_EDGE('',*,*,#15804,.F.);
#21158=ORIENTED_EDGE('',*,*,#15801,.F.);
#21159=ORIENTED_EDGE('',*,*,#15805,.T.);
#21160=ORIENTED_EDGE('',*,*,#15806,.T.);
#21161=ORIENTED_EDGE('',*,*,#15807,.T.);
#21162=ORIENTED_EDGE('',*,*,#15806,.F.);
#21163=ORIENTED_EDGE('',*,*,#15805,.F.);
#21164=ORIENTED_EDGE('',*,*,#15808,.T.);
#21165=ORIENTED_EDGE('',*,*,#15809,.F.);
#21166=ORIENTED_EDGE('',*,*,#15808,.F.);
#21167=ORIENTED_EDGE('',*,*,#15810,.F.);
#21168=ORIENTED_EDGE('',*,*,#15807,.F.);
#21169=ORIENTED_EDGE('',*,*,#15811,.T.);
#21170=ORIENTED_EDGE('',*,*,#15812,.T.);
#21171=ORIENTED_EDGE('',*,*,#15813,.T.);
#21172=ORIENTED_EDGE('',*,*,#15812,.F.);
#21173=ORIENTED_EDGE('',*,*,#15811,.F.);
#21174=ORIENTED_EDGE('',*,*,#15814,.T.);
#21175=ORIENTED_EDGE('',*,*,#15815,.F.);
#21176=ORIENTED_EDGE('',*,*,#15814,.F.);
#21177=ORIENTED_EDGE('',*,*,#15816,.F.);
#21178=ORIENTED_EDGE('',*,*,#15813,.F.);
#21179=ORIENTED_EDGE('',*,*,#15817,.T.);
#21180=ORIENTED_EDGE('',*,*,#15818,.T.);
#21181=ORIENTED_EDGE('',*,*,#15819,.T.);
#21182=ORIENTED_EDGE('',*,*,#15818,.F.);
#21183=ORIENTED_EDGE('',*,*,#15817,.F.);
#21184=ORIENTED_EDGE('',*,*,#15820,.T.);
#21185=ORIENTED_EDGE('',*,*,#15821,.F.);
#21186=ORIENTED_EDGE('',*,*,#15820,.F.);
#21187=ORIENTED_EDGE('',*,*,#15822,.F.);
#21188=ORIENTED_EDGE('',*,*,#15819,.F.);
#21189=ORIENTED_EDGE('',*,*,#15823,.T.);
#21190=ORIENTED_EDGE('',*,*,#15824,.T.);
#21191=ORIENTED_EDGE('',*,*,#15825,.T.);
#21192=ORIENTED_EDGE('',*,*,#15824,.F.);
#21193=ORIENTED_EDGE('',*,*,#15823,.F.);
#21194=ORIENTED_EDGE('',*,*,#15826,.T.);
#21195=ORIENTED_EDGE('',*,*,#15827,.F.);
#21196=ORIENTED_EDGE('',*,*,#15826,.F.);
#21197=ORIENTED_EDGE('',*,*,#15828,.F.);
#21198=ORIENTED_EDGE('',*,*,#15825,.F.);
#21199=ORIENTED_EDGE('',*,*,#15829,.T.);
#21200=ORIENTED_EDGE('',*,*,#15830,.T.);
#21201=ORIENTED_EDGE('',*,*,#15831,.T.);
#21202=ORIENTED_EDGE('',*,*,#15830,.F.);
#21203=ORIENTED_EDGE('',*,*,#15832,.F.);
#21204=ORIENTED_EDGE('',*,*,#15833,.T.);
#21205=ORIENTED_EDGE('',*,*,#15829,.F.);
#21206=ORIENTED_EDGE('',*,*,#15833,.F.);
#21207=ORIENTED_EDGE('',*,*,#15834,.F.);
#21208=ORIENTED_EDGE('',*,*,#15831,.F.);
#21209=ORIENTED_EDGE('',*,*,#15835,.T.);
#21210=ORIENTED_EDGE('',*,*,#15836,.T.);
#21211=ORIENTED_EDGE('',*,*,#15837,.T.);
#21212=ORIENTED_EDGE('',*,*,#15838,.T.);
#21213=ORIENTED_EDGE('',*,*,#15839,.T.);
#21214=ORIENTED_EDGE('',*,*,#15840,.T.);
#21215=ORIENTED_EDGE('',*,*,#15840,.F.);
#21216=ORIENTED_EDGE('',*,*,#15841,.T.);
#21217=ORIENTED_EDGE('',*,*,#15842,.F.);
#21218=ORIENTED_EDGE('',*,*,#15843,.F.);
#21219=ORIENTED_EDGE('',*,*,#15844,.T.);
#21220=ORIENTED_EDGE('',*,*,#15845,.T.);
#21221=ORIENTED_EDGE('',*,*,#15839,.F.);
#21222=ORIENTED_EDGE('',*,*,#15846,.F.);
#21223=ORIENTED_EDGE('',*,*,#15847,.F.);
#21224=ORIENTED_EDGE('',*,*,#15841,.F.);
#21225=ORIENTED_EDGE('',*,*,#15838,.F.);
#21226=ORIENTED_EDGE('',*,*,#15848,.F.);
#21227=ORIENTED_EDGE('',*,*,#15849,.T.);
#21228=ORIENTED_EDGE('',*,*,#15850,.T.);
#21229=ORIENTED_EDGE('',*,*,#15851,.F.);
#21230=ORIENTED_EDGE('',*,*,#15846,.T.);
#21231=ORIENTED_EDGE('',*,*,#15852,.T.);
#21232=ORIENTED_EDGE('',*,*,#15853,.T.);
#21233=ORIENTED_EDGE('',*,*,#15854,.T.);
#21234=ORIENTED_EDGE('',*,*,#15853,.F.);
#21235=ORIENTED_EDGE('',*,*,#15852,.F.);
#21236=ORIENTED_EDGE('',*,*,#15855,.T.);
#21237=ORIENTED_EDGE('',*,*,#15856,.F.);
#21238=ORIENTED_EDGE('',*,*,#15855,.F.);
#21239=ORIENTED_EDGE('',*,*,#15857,.F.);
#21240=ORIENTED_EDGE('',*,*,#15854,.F.);
#21241=ORIENTED_EDGE('',*,*,#15858,.T.);
#21242=ORIENTED_EDGE('',*,*,#15859,.T.);
#21243=ORIENTED_EDGE('',*,*,#15860,.T.);
#21244=ORIENTED_EDGE('',*,*,#15859,.F.);
#21245=ORIENTED_EDGE('',*,*,#15858,.F.);
#21246=ORIENTED_EDGE('',*,*,#15861,.T.);
#21247=ORIENTED_EDGE('',*,*,#15862,.F.);
#21248=ORIENTED_EDGE('',*,*,#15861,.F.);
#21249=ORIENTED_EDGE('',*,*,#15863,.F.);
#21250=ORIENTED_EDGE('',*,*,#15860,.F.);
#21251=ORIENTED_EDGE('',*,*,#15864,.T.);
#21252=ORIENTED_EDGE('',*,*,#15865,.T.);
#21253=ORIENTED_EDGE('',*,*,#15866,.T.);
#21254=ORIENTED_EDGE('',*,*,#15867,.T.);
#21255=ORIENTED_EDGE('',*,*,#15868,.T.);
#21256=ORIENTED_EDGE('',*,*,#15869,.T.);
#21257=ORIENTED_EDGE('',*,*,#15866,.F.);
#21258=ORIENTED_EDGE('',*,*,#15870,.T.);
#21259=ORIENTED_EDGE('',*,*,#15871,.F.);
#21260=ORIENTED_EDGE('',*,*,#15872,.T.);
#21261=ORIENTED_EDGE('',*,*,#15873,.T.);
#21262=ORIENTED_EDGE('',*,*,#15874,.T.);
#21263=ORIENTED_EDGE('',*,*,#15865,.F.);
#21264=ORIENTED_EDGE('',*,*,#15875,.F.);
#21265=ORIENTED_EDGE('',*,*,#15876,.F.);
#21266=ORIENTED_EDGE('',*,*,#15870,.F.);
#21267=ORIENTED_EDGE('',*,*,#15864,.F.);
#21268=ORIENTED_EDGE('',*,*,#15877,.F.);
#21269=ORIENTED_EDGE('',*,*,#15878,.T.);
#21270=ORIENTED_EDGE('',*,*,#15879,.T.);
#21271=ORIENTED_EDGE('',*,*,#15880,.F.);
#21272=ORIENTED_EDGE('',*,*,#15875,.T.);
#21273=ORIENTED_EDGE('',*,*,#15842,.T.);
#21274=ORIENTED_EDGE('',*,*,#15847,.T.);
#21275=ORIENTED_EDGE('',*,*,#15851,.T.);
#21276=ORIENTED_EDGE('',*,*,#15881,.T.);
#21277=ORIENTED_EDGE('',*,*,#15882,.T.);
#21278=ORIENTED_EDGE('',*,*,#15883,.T.);
#21279=ORIENTED_EDGE('',*,*,#15884,.T.);
#21280=ORIENTED_EDGE('',*,*,#15885,.T.);
#21281=ORIENTED_EDGE('',*,*,#15886,.T.);
#21282=ORIENTED_EDGE('',*,*,#15871,.T.);
#21283=ORIENTED_EDGE('',*,*,#15876,.T.);
#21284=ORIENTED_EDGE('',*,*,#15880,.T.);
#21285=ORIENTED_EDGE('',*,*,#15887,.T.);
#21286=ORIENTED_EDGE('',*,*,#15888,.T.);
#21287=ORIENTED_EDGE('',*,*,#15889,.T.);
#21288=ORIENTED_EDGE('',*,*,#15888,.F.);
#21289=ORIENTED_EDGE('',*,*,#15887,.F.);
#21290=ORIENTED_EDGE('',*,*,#15890,.T.);
#21291=ORIENTED_EDGE('',*,*,#15891,.F.);
#21292=ORIENTED_EDGE('',*,*,#15890,.F.);
#21293=ORIENTED_EDGE('',*,*,#15892,.F.);
#21294=ORIENTED_EDGE('',*,*,#15889,.F.);
#21295=ORIENTED_EDGE('',*,*,#15893,.T.);
#21296=ORIENTED_EDGE('',*,*,#15894,.T.);
#21297=ORIENTED_EDGE('',*,*,#15895,.T.);
#21298=ORIENTED_EDGE('',*,*,#15894,.F.);
#21299=ORIENTED_EDGE('',*,*,#15893,.F.);
#21300=ORIENTED_EDGE('',*,*,#15896,.T.);
#21301=ORIENTED_EDGE('',*,*,#15897,.F.);
#21302=ORIENTED_EDGE('',*,*,#15896,.F.);
#21303=ORIENTED_EDGE('',*,*,#15898,.F.);
#21304=ORIENTED_EDGE('',*,*,#15895,.F.);
#21305=ORIENTED_EDGE('',*,*,#15899,.T.);
#21306=ORIENTED_EDGE('',*,*,#15900,.T.);
#21307=ORIENTED_EDGE('',*,*,#15821,.T.);
#21308=ORIENTED_EDGE('',*,*,#15900,.F.);
#21309=ORIENTED_EDGE('',*,*,#15873,.F.);
#21310=ORIENTED_EDGE('',*,*,#15901,.F.);
#21311=ORIENTED_EDGE('',*,*,#15849,.F.);
#21312=ORIENTED_EDGE('',*,*,#15902,.F.);
#21313=ORIENTED_EDGE('',*,*,#15903,.F.);
#21314=ORIENTED_EDGE('',*,*,#15904,.F.);
#21315=ORIENTED_EDGE('',*,*,#15905,.F.);
#21316=ORIENTED_EDGE('',*,*,#15906,.F.);
#21317=ORIENTED_EDGE('',*,*,#15907,.F.);
#21318=ORIENTED_EDGE('',*,*,#15908,.F.);
#21319=ORIENTED_EDGE('',*,*,#15909,.F.);
#21320=ORIENTED_EDGE('',*,*,#15910,.F.);
#21321=ORIENTED_EDGE('',*,*,#15911,.F.);
#21322=ORIENTED_EDGE('',*,*,#15912,.F.);
#21323=ORIENTED_EDGE('',*,*,#15913,.F.);
#21324=ORIENTED_EDGE('',*,*,#15914,.F.);
#21325=ORIENTED_EDGE('',*,*,#15915,.F.);
#21326=ORIENTED_EDGE('',*,*,#15916,.F.);
#21327=ORIENTED_EDGE('',*,*,#15917,.F.);
#21328=ORIENTED_EDGE('',*,*,#15918,.F.);
#21329=ORIENTED_EDGE('',*,*,#15919,.F.);
#21330=ORIENTED_EDGE('',*,*,#15920,.F.);
#21331=ORIENTED_EDGE('',*,*,#15921,.F.);
#21332=ORIENTED_EDGE('',*,*,#15922,.F.);
#21333=ORIENTED_EDGE('',*,*,#15923,.F.);
#21334=ORIENTED_EDGE('',*,*,#15924,.T.);
#21335=ORIENTED_EDGE('',*,*,#15925,.F.);
#21336=ORIENTED_EDGE('',*,*,#15926,.F.);
#21337=ORIENTED_EDGE('',*,*,#15927,.F.);
#21338=ORIENTED_EDGE('',*,*,#15928,.F.);
#21339=ORIENTED_EDGE('',*,*,#15929,.F.);
#21340=ORIENTED_EDGE('',*,*,#15930,.F.);
#21341=ORIENTED_EDGE('',*,*,#15931,.F.);
#21342=ORIENTED_EDGE('',*,*,#15932,.F.);
#21343=ORIENTED_EDGE('',*,*,#15933,.F.);
#21344=ORIENTED_EDGE('',*,*,#15934,.F.);
#21345=ORIENTED_EDGE('',*,*,#15935,.F.);
#21346=ORIENTED_EDGE('',*,*,#15936,.F.);
#21347=ORIENTED_EDGE('',*,*,#15937,.F.);
#21348=ORIENTED_EDGE('',*,*,#15938,.F.);
#21349=ORIENTED_EDGE('',*,*,#15939,.F.);
#21350=ORIENTED_EDGE('',*,*,#15940,.F.);
#21351=ORIENTED_EDGE('',*,*,#15941,.F.);
#21352=ORIENTED_EDGE('',*,*,#15942,.F.);
#21353=ORIENTED_EDGE('',*,*,#15943,.F.);
#21354=ORIENTED_EDGE('',*,*,#15899,.F.);
#21355=ORIENTED_EDGE('',*,*,#15903,.T.);
#21356=ORIENTED_EDGE('',*,*,#15944,.T.);
#21357=ORIENTED_EDGE('',*,*,#15815,.T.);
#21358=ORIENTED_EDGE('',*,*,#15944,.F.);
#21359=ORIENTED_EDGE('',*,*,#15943,.T.);
#21360=ORIENTED_EDGE('',*,*,#15945,.T.);
#21361=ORIENTED_EDGE('',*,*,#15809,.T.);
#21362=ORIENTED_EDGE('',*,*,#15945,.F.);
#21363=ORIENTED_EDGE('',*,*,#15904,.T.);
#21364=ORIENTED_EDGE('',*,*,#15946,.T.);
#21365=ORIENTED_EDGE('',*,*,#15803,.T.);
#21366=ORIENTED_EDGE('',*,*,#15946,.F.);
#21367=ORIENTED_EDGE('',*,*,#15942,.T.);
#21368=ORIENTED_EDGE('',*,*,#15947,.T.);
#21369=ORIENTED_EDGE('',*,*,#15797,.T.);
#21370=ORIENTED_EDGE('',*,*,#15947,.F.);
#21371=ORIENTED_EDGE('',*,*,#15905,.T.);
#21372=ORIENTED_EDGE('',*,*,#15948,.T.);
#21373=ORIENTED_EDGE('',*,*,#15791,.T.);
#21374=ORIENTED_EDGE('',*,*,#15948,.F.);
#21375=ORIENTED_EDGE('',*,*,#15941,.T.);
#21376=ORIENTED_EDGE('',*,*,#15949,.T.);
#21377=ORIENTED_EDGE('',*,*,#15785,.T.);
#21378=ORIENTED_EDGE('',*,*,#15949,.F.);
#21379=ORIENTED_EDGE('',*,*,#15906,.T.);
#21380=ORIENTED_EDGE('',*,*,#15950,.T.);
#21381=ORIENTED_EDGE('',*,*,#15827,.T.);
#21382=ORIENTED_EDGE('',*,*,#15950,.F.);
#21383=ORIENTED_EDGE('',*,*,#15940,.T.);
#21384=ORIENTED_EDGE('',*,*,#15951,.T.);
#21385=ORIENTED_EDGE('',*,*,#15952,.T.);
#21386=ORIENTED_EDGE('',*,*,#15951,.F.);
#21387=ORIENTED_EDGE('',*,*,#15953,.F.);
#21388=ORIENTED_EDGE('',*,*,#15954,.T.);
#21389=ORIENTED_EDGE('',*,*,#15952,.F.);
#21390=ORIENTED_EDGE('',*,*,#15954,.F.);
#21391=ORIENTED_EDGE('',*,*,#15907,.T.);
#21392=ORIENTED_EDGE('',*,*,#15955,.T.);
#21393=ORIENTED_EDGE('',*,*,#15956,.T.);
#21394=ORIENTED_EDGE('',*,*,#15955,.F.);
#21395=ORIENTED_EDGE('',*,*,#15957,.F.);
#21396=ORIENTED_EDGE('',*,*,#15958,.T.);
#21397=ORIENTED_EDGE('',*,*,#15956,.F.);
#21398=ORIENTED_EDGE('',*,*,#15958,.F.);
#21399=ORIENTED_EDGE('',*,*,#15939,.T.);
#21400=ORIENTED_EDGE('',*,*,#15959,.T.);
#21401=ORIENTED_EDGE('',*,*,#15897,.T.);
#21402=ORIENTED_EDGE('',*,*,#15959,.F.);
#21403=ORIENTED_EDGE('',*,*,#15908,.T.);
#21404=ORIENTED_EDGE('',*,*,#15960,.T.);
#21405=ORIENTED_EDGE('',*,*,#15891,.T.);
#21406=ORIENTED_EDGE('',*,*,#15960,.F.);
#21407=ORIENTED_EDGE('',*,*,#15881,.F.);
#21408=ORIENTED_EDGE('',*,*,#15850,.F.);
#21409=ORIENTED_EDGE('',*,*,#15901,.T.);
#21410=ORIENTED_EDGE('',*,*,#15872,.F.);
#21411=ORIENTED_EDGE('',*,*,#15886,.F.);
#21412=ORIENTED_EDGE('',*,*,#15961,.T.);
#21413=ORIENTED_EDGE('',*,*,#15837,.F.);
#21414=ORIENTED_EDGE('',*,*,#15962,.T.);
#21415=ORIENTED_EDGE('',*,*,#15867,.F.);
#21416=ORIENTED_EDGE('',*,*,#15874,.F.);
#21417=ORIENTED_EDGE('',*,*,#15902,.T.);
#21418=ORIENTED_EDGE('',*,*,#15848,.T.);
#21419=ORIENTED_EDGE('',*,*,#15882,.F.);
#21420=ORIENTED_EDGE('',*,*,#15961,.F.);
#21421=ORIENTED_EDGE('',*,*,#15885,.F.);
#21422=ORIENTED_EDGE('',*,*,#15963,.F.);
#21423=ORIENTED_EDGE('',*,*,#15909,.T.);
#21424=ORIENTED_EDGE('',*,*,#15964,.T.);
#21425=ORIENTED_EDGE('',*,*,#15965,.T.);
#21426=ORIENTED_EDGE('',*,*,#15964,.F.);
#21427=ORIENTED_EDGE('',*,*,#15966,.F.);
#21428=ORIENTED_EDGE('',*,*,#15967,.T.);
#21429=ORIENTED_EDGE('',*,*,#15965,.F.);
#21430=ORIENTED_EDGE('',*,*,#15967,.F.);
#21431=ORIENTED_EDGE('',*,*,#15938,.T.);
#21432=ORIENTED_EDGE('',*,*,#15968,.T.);
#21433=ORIENTED_EDGE('',*,*,#15969,.T.);
#21434=ORIENTED_EDGE('',*,*,#15968,.F.);
#21435=ORIENTED_EDGE('',*,*,#15970,.F.);
#21436=ORIENTED_EDGE('',*,*,#15971,.T.);
#21437=ORIENTED_EDGE('',*,*,#15969,.F.);
#21438=ORIENTED_EDGE('',*,*,#15971,.F.);
#21439=ORIENTED_EDGE('',*,*,#15910,.T.);
#21440=ORIENTED_EDGE('',*,*,#15972,.T.);
#21441=ORIENTED_EDGE('',*,*,#15973,.T.);
#21442=ORIENTED_EDGE('',*,*,#15972,.F.);
#21443=ORIENTED_EDGE('',*,*,#15974,.F.);
#21444=ORIENTED_EDGE('',*,*,#15975,.T.);
#21445=ORIENTED_EDGE('',*,*,#15973,.F.);
#21446=ORIENTED_EDGE('',*,*,#15975,.F.);
#21447=ORIENTED_EDGE('',*,*,#15937,.T.);
#21448=ORIENTED_EDGE('',*,*,#15976,.T.);
#21449=ORIENTED_EDGE('',*,*,#15977,.T.);
#21450=ORIENTED_EDGE('',*,*,#15976,.F.);
#21451=ORIENTED_EDGE('',*,*,#15978,.F.);
#21452=ORIENTED_EDGE('',*,*,#15979,.T.);
#21453=ORIENTED_EDGE('',*,*,#15977,.F.);
#21454=ORIENTED_EDGE('',*,*,#15979,.F.);
#21455=ORIENTED_EDGE('',*,*,#15911,.T.);
#21456=ORIENTED_EDGE('',*,*,#15980,.T.);
#21457=ORIENTED_EDGE('',*,*,#15981,.T.);
#21458=ORIENTED_EDGE('',*,*,#15980,.F.);
#21459=ORIENTED_EDGE('',*,*,#15982,.F.);
#21460=ORIENTED_EDGE('',*,*,#15983,.T.);
#21461=ORIENTED_EDGE('',*,*,#15981,.F.);
#21462=ORIENTED_EDGE('',*,*,#15983,.F.);
#21463=ORIENTED_EDGE('',*,*,#15936,.T.);
#21464=ORIENTED_EDGE('',*,*,#15984,.T.);
#21465=ORIENTED_EDGE('',*,*,#15985,.T.);
#21466=ORIENTED_EDGE('',*,*,#15984,.F.);
#21467=ORIENTED_EDGE('',*,*,#15986,.F.);
#21468=ORIENTED_EDGE('',*,*,#15987,.T.);
#21469=ORIENTED_EDGE('',*,*,#15985,.F.);
#21470=ORIENTED_EDGE('',*,*,#15987,.F.);
#21471=ORIENTED_EDGE('',*,*,#15912,.T.);
#21472=ORIENTED_EDGE('',*,*,#15988,.T.);
#21473=ORIENTED_EDGE('',*,*,#15989,.T.);
#21474=ORIENTED_EDGE('',*,*,#15988,.F.);
#21475=ORIENTED_EDGE('',*,*,#15990,.F.);
#21476=ORIENTED_EDGE('',*,*,#15991,.T.);
#21477=ORIENTED_EDGE('',*,*,#15989,.F.);
#21478=ORIENTED_EDGE('',*,*,#15991,.F.);
#21479=ORIENTED_EDGE('',*,*,#15935,.T.);
#21480=ORIENTED_EDGE('',*,*,#15992,.T.);
#21481=ORIENTED_EDGE('',*,*,#15993,.T.);
#21482=ORIENTED_EDGE('',*,*,#15992,.F.);
#21483=ORIENTED_EDGE('',*,*,#15994,.F.);
#21484=ORIENTED_EDGE('',*,*,#15995,.T.);
#21485=ORIENTED_EDGE('',*,*,#15993,.F.);
#21486=ORIENTED_EDGE('',*,*,#15995,.F.);
#21487=ORIENTED_EDGE('',*,*,#15913,.T.);
#21488=ORIENTED_EDGE('',*,*,#15996,.T.);
#21489=ORIENTED_EDGE('',*,*,#15997,.T.);
#21490=ORIENTED_EDGE('',*,*,#15996,.F.);
#21491=ORIENTED_EDGE('',*,*,#15998,.F.);
#21492=ORIENTED_EDGE('',*,*,#15999,.T.);
#21493=ORIENTED_EDGE('',*,*,#15997,.F.);
#21494=ORIENTED_EDGE('',*,*,#15999,.F.);
#21495=ORIENTED_EDGE('',*,*,#15934,.T.);
#21496=ORIENTED_EDGE('',*,*,#16000,.T.);
#21497=ORIENTED_EDGE('',*,*,#16001,.T.);
#21498=ORIENTED_EDGE('',*,*,#16000,.F.);
#21499=ORIENTED_EDGE('',*,*,#16002,.F.);
#21500=ORIENTED_EDGE('',*,*,#16003,.T.);
#21501=ORIENTED_EDGE('',*,*,#16001,.F.);
#21502=ORIENTED_EDGE('',*,*,#16003,.F.);
#21503=ORIENTED_EDGE('',*,*,#15914,.T.);
#21504=ORIENTED_EDGE('',*,*,#16004,.T.);
#21505=ORIENTED_EDGE('',*,*,#16005,.T.);
#21506=ORIENTED_EDGE('',*,*,#16004,.F.);
#21507=ORIENTED_EDGE('',*,*,#16006,.F.);
#21508=ORIENTED_EDGE('',*,*,#16007,.T.);
#21509=ORIENTED_EDGE('',*,*,#16005,.F.);
#21510=ORIENTED_EDGE('',*,*,#16007,.F.);
#21511=ORIENTED_EDGE('',*,*,#15933,.T.);
#21512=ORIENTED_EDGE('',*,*,#16008,.T.);
#21513=ORIENTED_EDGE('',*,*,#16009,.T.);
#21514=ORIENTED_EDGE('',*,*,#16008,.F.);
#21515=ORIENTED_EDGE('',*,*,#16010,.F.);
#21516=ORIENTED_EDGE('',*,*,#16011,.T.);
#21517=ORIENTED_EDGE('',*,*,#16009,.F.);
#21518=ORIENTED_EDGE('',*,*,#16011,.F.);
#21519=ORIENTED_EDGE('',*,*,#15915,.T.);
#21520=ORIENTED_EDGE('',*,*,#16012,.T.);
#21521=ORIENTED_EDGE('',*,*,#15862,.T.);
#21522=ORIENTED_EDGE('',*,*,#16012,.F.);
#21523=ORIENTED_EDGE('',*,*,#15932,.T.);
#21524=ORIENTED_EDGE('',*,*,#16013,.T.);
#21525=ORIENTED_EDGE('',*,*,#15856,.T.);
#21526=ORIENTED_EDGE('',*,*,#16013,.F.);
#21527=ORIENTED_EDGE('',*,*,#15916,.T.);
#21528=ORIENTED_EDGE('',*,*,#16014,.T.);
#21529=ORIENTED_EDGE('',*,*,#16015,.T.);
#21530=ORIENTED_EDGE('',*,*,#16014,.F.);
#21531=ORIENTED_EDGE('',*,*,#16016,.F.);
#21532=ORIENTED_EDGE('',*,*,#16017,.T.);
#21533=ORIENTED_EDGE('',*,*,#16015,.F.);
#21534=ORIENTED_EDGE('',*,*,#16017,.F.);
#21535=ORIENTED_EDGE('',*,*,#15931,.T.);
#21536=ORIENTED_EDGE('',*,*,#16018,.T.);
#21537=ORIENTED_EDGE('',*,*,#16019,.T.);
#21538=ORIENTED_EDGE('',*,*,#16018,.F.);
#21539=ORIENTED_EDGE('',*,*,#16020,.F.);
#21540=ORIENTED_EDGE('',*,*,#16021,.T.);
#21541=ORIENTED_EDGE('',*,*,#16019,.F.);
#21542=ORIENTED_EDGE('',*,*,#16021,.F.);
#21543=ORIENTED_EDGE('',*,*,#15917,.T.);
#21544=ORIENTED_EDGE('',*,*,#16022,.T.);
#21545=ORIENTED_EDGE('',*,*,#16023,.T.);
#21546=ORIENTED_EDGE('',*,*,#16022,.F.);
#21547=ORIENTED_EDGE('',*,*,#16024,.F.);
#21548=ORIENTED_EDGE('',*,*,#16025,.T.);
#21549=ORIENTED_EDGE('',*,*,#16023,.F.);
#21550=ORIENTED_EDGE('',*,*,#16025,.F.);
#21551=ORIENTED_EDGE('',*,*,#15930,.T.);
#21552=ORIENTED_EDGE('',*,*,#16026,.T.);
#21553=ORIENTED_EDGE('',*,*,#16027,.T.);
#21554=ORIENTED_EDGE('',*,*,#16026,.F.);
#21555=ORIENTED_EDGE('',*,*,#16028,.F.);
#21556=ORIENTED_EDGE('',*,*,#16029,.T.);
#21557=ORIENTED_EDGE('',*,*,#16027,.F.);
#21558=ORIENTED_EDGE('',*,*,#16029,.F.);
#21559=ORIENTED_EDGE('',*,*,#15918,.T.);
#21560=ORIENTED_EDGE('',*,*,#16030,.T.);
#21561=ORIENTED_EDGE('',*,*,#16031,.T.);
#21562=ORIENTED_EDGE('',*,*,#16030,.F.);
#21563=ORIENTED_EDGE('',*,*,#16032,.F.);
#21564=ORIENTED_EDGE('',*,*,#16033,.T.);
#21565=ORIENTED_EDGE('',*,*,#16031,.F.);
#21566=ORIENTED_EDGE('',*,*,#16033,.F.);
#21567=ORIENTED_EDGE('',*,*,#15929,.T.);
#21568=ORIENTED_EDGE('',*,*,#16034,.T.);
#21569=ORIENTED_EDGE('',*,*,#16035,.T.);
#21570=ORIENTED_EDGE('',*,*,#16034,.F.);
#21571=ORIENTED_EDGE('',*,*,#16036,.F.);
#21572=ORIENTED_EDGE('',*,*,#16037,.T.);
#21573=ORIENTED_EDGE('',*,*,#16035,.F.);
#21574=ORIENTED_EDGE('',*,*,#16037,.F.);
#21575=ORIENTED_EDGE('',*,*,#15919,.T.);
#21576=ORIENTED_EDGE('',*,*,#16038,.T.);
#21577=ORIENTED_EDGE('',*,*,#16039,.T.);
#21578=ORIENTED_EDGE('',*,*,#16038,.F.);
#21579=ORIENTED_EDGE('',*,*,#16040,.F.);
#21580=ORIENTED_EDGE('',*,*,#16041,.T.);
#21581=ORIENTED_EDGE('',*,*,#16039,.F.);
#21582=ORIENTED_EDGE('',*,*,#16041,.F.);
#21583=ORIENTED_EDGE('',*,*,#15928,.T.);
#21584=ORIENTED_EDGE('',*,*,#16042,.T.);
#21585=ORIENTED_EDGE('',*,*,#16043,.T.);
#21586=ORIENTED_EDGE('',*,*,#16042,.F.);
#21587=ORIENTED_EDGE('',*,*,#16044,.F.);
#21588=ORIENTED_EDGE('',*,*,#16045,.T.);
#21589=ORIENTED_EDGE('',*,*,#16043,.F.);
#21590=ORIENTED_EDGE('',*,*,#16045,.F.);
#21591=ORIENTED_EDGE('',*,*,#15920,.T.);
#21592=ORIENTED_EDGE('',*,*,#16046,.T.);
#21593=ORIENTED_EDGE('',*,*,#16047,.T.);
#21594=ORIENTED_EDGE('',*,*,#16046,.F.);
#21595=ORIENTED_EDGE('',*,*,#16048,.F.);
#21596=ORIENTED_EDGE('',*,*,#16049,.T.);
#21597=ORIENTED_EDGE('',*,*,#16047,.F.);
#21598=ORIENTED_EDGE('',*,*,#16049,.F.);
#21599=ORIENTED_EDGE('',*,*,#15927,.T.);
#21600=ORIENTED_EDGE('',*,*,#16050,.T.);
#21601=ORIENTED_EDGE('',*,*,#16051,.T.);
#21602=ORIENTED_EDGE('',*,*,#16050,.F.);
#21603=ORIENTED_EDGE('',*,*,#16052,.F.);
#21604=ORIENTED_EDGE('',*,*,#16053,.T.);
#21605=ORIENTED_EDGE('',*,*,#16051,.F.);
#21606=ORIENTED_EDGE('',*,*,#16053,.F.);
#21607=ORIENTED_EDGE('',*,*,#15921,.T.);
#21608=ORIENTED_EDGE('',*,*,#16054,.T.);
#21609=ORIENTED_EDGE('',*,*,#16055,.T.);
#21610=ORIENTED_EDGE('',*,*,#16054,.F.);
#21611=ORIENTED_EDGE('',*,*,#16056,.F.);
#21612=ORIENTED_EDGE('',*,*,#16057,.T.);
#21613=ORIENTED_EDGE('',*,*,#16055,.F.);
#21614=ORIENTED_EDGE('',*,*,#16057,.F.);
#21615=ORIENTED_EDGE('',*,*,#15926,.T.);
#21616=ORIENTED_EDGE('',*,*,#16058,.T.);
#21617=ORIENTED_EDGE('',*,*,#16059,.T.);
#21618=ORIENTED_EDGE('',*,*,#16058,.F.);
#21619=ORIENTED_EDGE('',*,*,#16060,.F.);
#21620=ORIENTED_EDGE('',*,*,#16061,.T.);
#21621=ORIENTED_EDGE('',*,*,#16059,.F.);
#21622=ORIENTED_EDGE('',*,*,#16061,.F.);
#21623=ORIENTED_EDGE('',*,*,#15922,.T.);
#21624=ORIENTED_EDGE('',*,*,#16062,.T.);
#21625=ORIENTED_EDGE('',*,*,#16063,.T.);
#21626=ORIENTED_EDGE('',*,*,#16062,.F.);
#21627=ORIENTED_EDGE('',*,*,#16064,.F.);
#21628=ORIENTED_EDGE('',*,*,#16065,.T.);
#21629=ORIENTED_EDGE('',*,*,#16063,.F.);
#21630=ORIENTED_EDGE('',*,*,#16065,.F.);
#21631=ORIENTED_EDGE('',*,*,#15925,.T.);
#21632=ORIENTED_EDGE('',*,*,#16066,.T.);
#21633=ORIENTED_EDGE('',*,*,#16067,.T.);
#21634=ORIENTED_EDGE('',*,*,#16066,.F.);
#21635=ORIENTED_EDGE('',*,*,#16068,.F.);
#21636=ORIENTED_EDGE('',*,*,#16069,.T.);
#21637=ORIENTED_EDGE('',*,*,#16067,.F.);
#21638=ORIENTED_EDGE('',*,*,#16069,.F.);
#21639=ORIENTED_EDGE('',*,*,#15923,.T.);
#21640=ORIENTED_EDGE('',*,*,#16070,.T.);
#21641=ORIENTED_EDGE('',*,*,#16071,.T.);
#21642=ORIENTED_EDGE('',*,*,#16070,.F.);
#21643=ORIENTED_EDGE('',*,*,#16072,.F.);
#21644=ORIENTED_EDGE('',*,*,#16073,.T.);
#21645=ORIENTED_EDGE('',*,*,#16071,.F.);
#21646=ORIENTED_EDGE('',*,*,#16073,.F.);
#21647=ORIENTED_EDGE('',*,*,#15835,.F.);
#21648=ORIENTED_EDGE('',*,*,#15845,.F.);
#21649=ORIENTED_EDGE('',*,*,#16074,.T.);
#21650=ORIENTED_EDGE('',*,*,#15877,.T.);
#21651=ORIENTED_EDGE('',*,*,#15869,.F.);
#21652=ORIENTED_EDGE('',*,*,#16075,.T.);
#21653=ORIENTED_EDGE('',*,*,#15883,.F.);
#21654=ORIENTED_EDGE('',*,*,#15963,.T.);
#21655=ORIENTED_EDGE('',*,*,#15884,.F.);
#21656=ORIENTED_EDGE('',*,*,#15879,.F.);
#21657=ORIENTED_EDGE('',*,*,#16076,.T.);
#21658=ORIENTED_EDGE('',*,*,#15843,.T.);
#21659=ORIENTED_EDGE('',*,*,#15844,.F.);
#21660=ORIENTED_EDGE('',*,*,#16076,.F.);
#21661=ORIENTED_EDGE('',*,*,#15878,.F.);
#21662=ORIENTED_EDGE('',*,*,#16074,.F.);
#21663=ORIENTED_EDGE('',*,*,#16077,.F.);
#21664=ORIENTED_EDGE('',*,*,#16078,.F.);
#21665=ORIENTED_EDGE('',*,*,#16079,.F.);
#21666=ORIENTED_EDGE('',*,*,#16080,.F.);
#21667=ORIENTED_EDGE('',*,*,#16081,.F.);
#21668=ORIENTED_EDGE('',*,*,#16082,.F.);
#21669=ORIENTED_EDGE('',*,*,#16083,.F.);
#21670=ORIENTED_EDGE('',*,*,#16084,.F.);
#21671=ORIENTED_EDGE('',*,*,#16085,.F.);
#21672=ORIENTED_EDGE('',*,*,#16086,.F.);
#21673=ORIENTED_EDGE('',*,*,#16087,.F.);
#21674=ORIENTED_EDGE('',*,*,#16088,.F.);
#21675=ORIENTED_EDGE('',*,*,#16089,.F.);
#21676=ORIENTED_EDGE('',*,*,#16090,.F.);
#21677=ORIENTED_EDGE('',*,*,#16091,.F.);
#21678=ORIENTED_EDGE('',*,*,#16092,.F.);
#21679=ORIENTED_EDGE('',*,*,#16093,.F.);
#21680=ORIENTED_EDGE('',*,*,#16094,.F.);
#21681=ORIENTED_EDGE('',*,*,#16095,.F.);
#21682=ORIENTED_EDGE('',*,*,#16096,.F.);
#21683=ORIENTED_EDGE('',*,*,#16097,.F.);
#21684=ORIENTED_EDGE('',*,*,#16098,.F.);
#21685=ORIENTED_EDGE('',*,*,#16099,.F.);
#21686=ORIENTED_EDGE('',*,*,#16100,.F.);
#21687=ORIENTED_EDGE('',*,*,#16101,.F.);
#21688=ORIENTED_EDGE('',*,*,#16102,.F.);
#21689=ORIENTED_EDGE('',*,*,#16103,.F.);
#21690=ORIENTED_EDGE('',*,*,#16104,.F.);
#21691=ORIENTED_EDGE('',*,*,#16105,.F.);
#21692=ORIENTED_EDGE('',*,*,#16106,.F.);
#21693=ORIENTED_EDGE('',*,*,#16107,.F.);
#21694=ORIENTED_EDGE('',*,*,#16108,.F.);
#21695=ORIENTED_EDGE('',*,*,#16109,.F.);
#21696=ORIENTED_EDGE('',*,*,#16110,.F.);
#21697=ORIENTED_EDGE('',*,*,#16111,.F.);
#21698=ORIENTED_EDGE('',*,*,#16112,.F.);
#21699=ORIENTED_EDGE('',*,*,#16113,.F.);
#21700=ORIENTED_EDGE('',*,*,#16114,.F.);
#21701=ORIENTED_EDGE('',*,*,#16115,.F.);
#21702=ORIENTED_EDGE('',*,*,#16116,.F.);
#21703=ORIENTED_EDGE('',*,*,#16117,.F.);
#21704=ORIENTED_EDGE('',*,*,#16118,.F.);
#21705=ORIENTED_EDGE('',*,*,#16077,.T.);
#21706=ORIENTED_EDGE('',*,*,#16119,.T.);
#21707=ORIENTED_EDGE('',*,*,#15832,.T.);
#21708=ORIENTED_EDGE('',*,*,#16119,.F.);
#21709=ORIENTED_EDGE('',*,*,#16118,.T.);
#21710=ORIENTED_EDGE('',*,*,#16120,.T.);
#21711=ORIENTED_EDGE('',*,*,#16072,.T.);
#21712=ORIENTED_EDGE('',*,*,#16120,.F.);
#21713=ORIENTED_EDGE('',*,*,#16078,.T.);
#21714=ORIENTED_EDGE('',*,*,#16121,.T.);
#21715=ORIENTED_EDGE('',*,*,#16068,.T.);
#21716=ORIENTED_EDGE('',*,*,#16121,.F.);
#21717=ORIENTED_EDGE('',*,*,#16117,.T.);
#21718=ORIENTED_EDGE('',*,*,#16122,.T.);
#21719=ORIENTED_EDGE('',*,*,#16064,.T.);
#21720=ORIENTED_EDGE('',*,*,#16122,.F.);
#21721=ORIENTED_EDGE('',*,*,#16079,.T.);
#21722=ORIENTED_EDGE('',*,*,#16123,.T.);
#21723=ORIENTED_EDGE('',*,*,#16060,.T.);
#21724=ORIENTED_EDGE('',*,*,#16123,.F.);
#21725=ORIENTED_EDGE('',*,*,#16116,.T.);
#21726=ORIENTED_EDGE('',*,*,#16124,.T.);
#21727=ORIENTED_EDGE('',*,*,#16056,.T.);
#21728=ORIENTED_EDGE('',*,*,#16124,.F.);
#21729=ORIENTED_EDGE('',*,*,#16080,.T.);
#21730=ORIENTED_EDGE('',*,*,#16125,.T.);
#21731=ORIENTED_EDGE('',*,*,#16052,.T.);
#21732=ORIENTED_EDGE('',*,*,#16125,.F.);
#21733=ORIENTED_EDGE('',*,*,#16115,.T.);
#21734=ORIENTED_EDGE('',*,*,#16126,.T.);
#21735=ORIENTED_EDGE('',*,*,#16048,.T.);
#21736=ORIENTED_EDGE('',*,*,#16126,.F.);
#21737=ORIENTED_EDGE('',*,*,#16081,.T.);
#21738=ORIENTED_EDGE('',*,*,#16127,.T.);
#21739=ORIENTED_EDGE('',*,*,#16128,.T.);
#21740=ORIENTED_EDGE('',*,*,#16127,.F.);
#21741=ORIENTED_EDGE('',*,*,#16128,.F.);
#21742=ORIENTED_EDGE('',*,*,#16129,.T.);
#21743=ORIENTED_EDGE('',*,*,#15892,.T.);
#21744=ORIENTED_EDGE('',*,*,#16129,.F.);
#21745=ORIENTED_EDGE('',*,*,#16114,.T.);
#21746=ORIENTED_EDGE('',*,*,#16130,.T.);
#21747=ORIENTED_EDGE('',*,*,#16131,.T.);
#21748=ORIENTED_EDGE('',*,*,#16130,.F.);
#21749=ORIENTED_EDGE('',*,*,#16131,.F.);
#21750=ORIENTED_EDGE('',*,*,#16132,.T.);
#21751=ORIENTED_EDGE('',*,*,#15898,.T.);
#21752=ORIENTED_EDGE('',*,*,#16132,.F.);
#21753=ORIENTED_EDGE('',*,*,#16082,.T.);
#21754=ORIENTED_EDGE('',*,*,#16133,.T.);
#21755=ORIENTED_EDGE('',*,*,#16134,.T.);
#21756=ORIENTED_EDGE('',*,*,#16133,.F.);
#21757=ORIENTED_EDGE('',*,*,#16134,.F.);
#21758=ORIENTED_EDGE('',*,*,#16135,.T.);
#21759=ORIENTED_EDGE('',*,*,#15822,.T.);
#21760=ORIENTED_EDGE('',*,*,#16135,.F.);
#21761=ORIENTED_EDGE('',*,*,#16113,.T.);
#21762=ORIENTED_EDGE('',*,*,#16136,.T.);
#21763=ORIENTED_EDGE('',*,*,#16137,.T.);
#21764=ORIENTED_EDGE('',*,*,#16136,.F.);
#21765=ORIENTED_EDGE('',*,*,#16137,.F.);
#21766=ORIENTED_EDGE('',*,*,#16138,.T.);
#21767=ORIENTED_EDGE('',*,*,#15816,.T.);
#21768=ORIENTED_EDGE('',*,*,#16138,.F.);
#21769=ORIENTED_EDGE('',*,*,#16083,.T.);
#21770=ORIENTED_EDGE('',*,*,#16139,.T.);
#21771=ORIENTED_EDGE('',*,*,#16140,.T.);
#21772=ORIENTED_EDGE('',*,*,#16139,.F.);
#21773=ORIENTED_EDGE('',*,*,#16140,.F.);
#21774=ORIENTED_EDGE('',*,*,#16141,.T.);
#21775=ORIENTED_EDGE('',*,*,#15810,.T.);
#21776=ORIENTED_EDGE('',*,*,#16141,.F.);
#21777=ORIENTED_EDGE('',*,*,#16112,.T.);
#21778=ORIENTED_EDGE('',*,*,#16142,.T.);
#21779=ORIENTED_EDGE('',*,*,#16143,.T.);
#21780=ORIENTED_EDGE('',*,*,#16142,.F.);
#21781=ORIENTED_EDGE('',*,*,#16143,.F.);
#21782=ORIENTED_EDGE('',*,*,#16144,.T.);
#21783=ORIENTED_EDGE('',*,*,#15804,.T.);
#21784=ORIENTED_EDGE('',*,*,#16144,.F.);
#21785=ORIENTED_EDGE('',*,*,#16084,.T.);
#21786=ORIENTED_EDGE('',*,*,#16145,.T.);
#21787=ORIENTED_EDGE('',*,*,#16146,.T.);
#21788=ORIENTED_EDGE('',*,*,#16145,.F.);
#21789=ORIENTED_EDGE('',*,*,#16146,.F.);
#21790=ORIENTED_EDGE('',*,*,#16147,.T.);
#21791=ORIENTED_EDGE('',*,*,#15798,.T.);
#21792=ORIENTED_EDGE('',*,*,#16147,.F.);
#21793=ORIENTED_EDGE('',*,*,#16111,.T.);
#21794=ORIENTED_EDGE('',*,*,#16148,.T.);
#21795=ORIENTED_EDGE('',*,*,#16149,.T.);
#21796=ORIENTED_EDGE('',*,*,#16148,.F.);
#21797=ORIENTED_EDGE('',*,*,#16149,.F.);
#21798=ORIENTED_EDGE('',*,*,#16150,.T.);
#21799=ORIENTED_EDGE('',*,*,#15792,.T.);
#21800=ORIENTED_EDGE('',*,*,#16150,.F.);
#21801=ORIENTED_EDGE('',*,*,#16085,.T.);
#21802=ORIENTED_EDGE('',*,*,#16151,.T.);
#21803=ORIENTED_EDGE('',*,*,#16152,.T.);
#21804=ORIENTED_EDGE('',*,*,#16151,.F.);
#21805=ORIENTED_EDGE('',*,*,#16152,.F.);
#21806=ORIENTED_EDGE('',*,*,#16153,.T.);
#21807=ORIENTED_EDGE('',*,*,#15786,.T.);
#21808=ORIENTED_EDGE('',*,*,#16153,.F.);
#21809=ORIENTED_EDGE('',*,*,#16110,.T.);
#21810=ORIENTED_EDGE('',*,*,#16154,.T.);
#21811=ORIENTED_EDGE('',*,*,#16155,.T.);
#21812=ORIENTED_EDGE('',*,*,#16154,.F.);
#21813=ORIENTED_EDGE('',*,*,#16155,.F.);
#21814=ORIENTED_EDGE('',*,*,#16156,.T.);
#21815=ORIENTED_EDGE('',*,*,#15828,.T.);
#21816=ORIENTED_EDGE('',*,*,#16156,.F.);
#21817=ORIENTED_EDGE('',*,*,#16086,.T.);
#21818=ORIENTED_EDGE('',*,*,#16157,.T.);
#21819=ORIENTED_EDGE('',*,*,#16044,.T.);
#21820=ORIENTED_EDGE('',*,*,#16157,.F.);
#21821=ORIENTED_EDGE('',*,*,#16109,.T.);
#21822=ORIENTED_EDGE('',*,*,#16158,.T.);
#21823=ORIENTED_EDGE('',*,*,#16040,.T.);
#21824=ORIENTED_EDGE('',*,*,#16158,.F.);
#21825=ORIENTED_EDGE('',*,*,#16087,.T.);
#21826=ORIENTED_EDGE('',*,*,#16159,.T.);
#21827=ORIENTED_EDGE('',*,*,#16036,.T.);
#21828=ORIENTED_EDGE('',*,*,#16159,.F.);
#21829=ORIENTED_EDGE('',*,*,#16108,.T.);
#21830=ORIENTED_EDGE('',*,*,#16160,.T.);
#21831=ORIENTED_EDGE('',*,*,#16032,.T.);
#21832=ORIENTED_EDGE('',*,*,#16160,.F.);
#21833=ORIENTED_EDGE('',*,*,#16088,.T.);
#21834=ORIENTED_EDGE('',*,*,#16161,.T.);
#21835=ORIENTED_EDGE('',*,*,#16028,.T.);
#21836=ORIENTED_EDGE('',*,*,#16161,.F.);
#21837=ORIENTED_EDGE('',*,*,#16107,.T.);
#21838=ORIENTED_EDGE('',*,*,#16162,.T.);
#21839=ORIENTED_EDGE('',*,*,#16024,.T.);
#21840=ORIENTED_EDGE('',*,*,#16162,.F.);
#21841=ORIENTED_EDGE('',*,*,#16089,.T.);
#21842=ORIENTED_EDGE('',*,*,#16163,.T.);
#21843=ORIENTED_EDGE('',*,*,#16020,.T.);
#21844=ORIENTED_EDGE('',*,*,#16163,.F.);
#21845=ORIENTED_EDGE('',*,*,#16106,.T.);
#21846=ORIENTED_EDGE('',*,*,#16164,.T.);
#21847=ORIENTED_EDGE('',*,*,#16016,.T.);
#21848=ORIENTED_EDGE('',*,*,#16164,.F.);
#21849=ORIENTED_EDGE('',*,*,#16090,.T.);
#21850=ORIENTED_EDGE('',*,*,#16165,.T.);
#21851=ORIENTED_EDGE('',*,*,#15966,.T.);
#21852=ORIENTED_EDGE('',*,*,#16165,.F.);
#21853=ORIENTED_EDGE('',*,*,#16105,.T.);
#21854=ORIENTED_EDGE('',*,*,#16166,.T.);
#21855=ORIENTED_EDGE('',*,*,#15970,.T.);
#21856=ORIENTED_EDGE('',*,*,#16166,.F.);
#21857=ORIENTED_EDGE('',*,*,#16091,.T.);
#21858=ORIENTED_EDGE('',*,*,#16167,.T.);
#21859=ORIENTED_EDGE('',*,*,#15974,.T.);
#21860=ORIENTED_EDGE('',*,*,#16167,.F.);
#21861=ORIENTED_EDGE('',*,*,#16104,.T.);
#21862=ORIENTED_EDGE('',*,*,#16168,.T.);
#21863=ORIENTED_EDGE('',*,*,#15978,.T.);
#21864=ORIENTED_EDGE('',*,*,#16168,.F.);
#21865=ORIENTED_EDGE('',*,*,#16092,.T.);
#21866=ORIENTED_EDGE('',*,*,#16169,.T.);
#21867=ORIENTED_EDGE('',*,*,#15982,.T.);
#21868=ORIENTED_EDGE('',*,*,#16169,.F.);
#21869=ORIENTED_EDGE('',*,*,#16103,.T.);
#21870=ORIENTED_EDGE('',*,*,#16170,.T.);
#21871=ORIENTED_EDGE('',*,*,#15986,.T.);
#21872=ORIENTED_EDGE('',*,*,#16170,.F.);
#21873=ORIENTED_EDGE('',*,*,#16093,.T.);
#21874=ORIENTED_EDGE('',*,*,#16171,.T.);
#21875=ORIENTED_EDGE('',*,*,#15990,.T.);
#21876=ORIENTED_EDGE('',*,*,#16171,.F.);
#21877=ORIENTED_EDGE('',*,*,#16102,.T.);
#21878=ORIENTED_EDGE('',*,*,#16172,.T.);
#21879=ORIENTED_EDGE('',*,*,#15994,.T.);
#21880=ORIENTED_EDGE('',*,*,#16172,.F.);
#21881=ORIENTED_EDGE('',*,*,#16094,.T.);
#21882=ORIENTED_EDGE('',*,*,#16173,.T.);
#21883=ORIENTED_EDGE('',*,*,#15998,.T.);
#21884=ORIENTED_EDGE('',*,*,#16173,.F.);
#21885=ORIENTED_EDGE('',*,*,#16101,.T.);
#21886=ORIENTED_EDGE('',*,*,#16174,.T.);
#21887=ORIENTED_EDGE('',*,*,#16002,.T.);
#21888=ORIENTED_EDGE('',*,*,#16174,.F.);
#21889=ORIENTED_EDGE('',*,*,#16095,.T.);
#21890=ORIENTED_EDGE('',*,*,#16175,.T.);
#21891=ORIENTED_EDGE('',*,*,#16006,.T.);
#21892=ORIENTED_EDGE('',*,*,#16175,.F.);
#21893=ORIENTED_EDGE('',*,*,#16100,.T.);
#21894=ORIENTED_EDGE('',*,*,#16176,.T.);
#21895=ORIENTED_EDGE('',*,*,#16010,.T.);
#21896=ORIENTED_EDGE('',*,*,#16176,.F.);
#21897=ORIENTED_EDGE('',*,*,#16096,.T.);
#21898=ORIENTED_EDGE('',*,*,#16177,.T.);
#21899=ORIENTED_EDGE('',*,*,#15953,.T.);
#21900=ORIENTED_EDGE('',*,*,#16177,.F.);
#21901=ORIENTED_EDGE('',*,*,#16099,.T.);
#21902=ORIENTED_EDGE('',*,*,#16178,.T.);
#21903=ORIENTED_EDGE('',*,*,#15957,.T.);
#21904=ORIENTED_EDGE('',*,*,#16178,.F.);
#21905=ORIENTED_EDGE('',*,*,#16097,.T.);
#21906=ORIENTED_EDGE('',*,*,#16179,.T.);
#21907=ORIENTED_EDGE('',*,*,#16180,.T.);
#21908=ORIENTED_EDGE('',*,*,#16179,.F.);
#21909=ORIENTED_EDGE('',*,*,#16180,.F.);
#21910=ORIENTED_EDGE('',*,*,#16181,.T.);
#21911=ORIENTED_EDGE('',*,*,#15863,.T.);
#21912=ORIENTED_EDGE('',*,*,#16181,.F.);
#21913=ORIENTED_EDGE('',*,*,#16098,.T.);
#21914=ORIENTED_EDGE('',*,*,#16182,.T.);
#21915=ORIENTED_EDGE('',*,*,#16183,.T.);
#21916=ORIENTED_EDGE('',*,*,#16182,.F.);
#21917=ORIENTED_EDGE('',*,*,#16183,.F.);
#21918=ORIENTED_EDGE('',*,*,#16184,.T.);
#21919=ORIENTED_EDGE('',*,*,#15857,.T.);
#21920=ORIENTED_EDGE('',*,*,#16184,.F.);
#21921=ORIENTED_EDGE('',*,*,#15924,.F.);
#21922=ORIENTED_EDGE('',*,*,#16185,.T.);
#21923=ORIENTED_EDGE('',*,*,#15834,.T.);
#21924=ORIENTED_EDGE('',*,*,#16185,.F.);
#21925=ORIENTED_EDGE('',*,*,#15836,.F.);
#21926=ORIENTED_EDGE('',*,*,#16075,.F.);
#21927=ORIENTED_EDGE('',*,*,#15868,.F.);
#21928=ORIENTED_EDGE('',*,*,#15962,.F.);
#28252=PLANE('',#31327);
#28253=PLANE('',#31334);
#28254=PLANE('',#31341);
#28255=PLANE('',#31348);
#28256=PLANE('',#31355);
#28257=PLANE('',#31362);
#28258=PLANE('',#31369);
#28259=PLANE('',#31376);
#28260=PLANE('',#31383);
#28261=PLANE('',#31385);
#28262=PLANE('',#31386);
#28263=PLANE('',#31387);
#28264=PLANE('',#31388);
#28265=PLANE('',#31394);
#28266=PLANE('',#31401);
#28267=PLANE('',#31403);
#28268=PLANE('',#31404);
#28269=PLANE('',#31405);
#28270=PLANE('',#31406);
#28271=PLANE('',#31407);
#28272=PLANE('',#31408);
#28273=PLANE('',#31414);
#28274=PLANE('',#31421);
#28275=PLANE('',#31425);
#28276=PLANE('',#31484);
#28277=PLANE('',#31485);
#28278=PLANE('',#31486);
#28279=PLANE('',#31597);
#28280=PLANE('',#31598);
#28281=PLANE('',#31599);
#28282=PLANE('',#31709);
#29283=ADVANCED_FACE('',(#3955),#1933,.F.);
#29284=ADVANCED_FACE('',(#3956),#483,.F.);
#29285=ADVANCED_FACE('',(#3957,#3337),#28252,.T.);
#29286=ADVANCED_FACE('',(#3958),#1934,.F.);
#29287=ADVANCED_FACE('',(#3959),#484,.F.);
#29288=ADVANCED_FACE('',(#3960,#3338),#28253,.T.);
#29289=ADVANCED_FACE('',(#3961),#1935,.F.);
#29290=ADVANCED_FACE('',(#3962),#485,.F.);
#29291=ADVANCED_FACE('',(#3963,#3339),#28254,.T.);
#29292=ADVANCED_FACE('',(#3964),#1936,.F.);
#29293=ADVANCED_FACE('',(#3965),#486,.F.);
#29294=ADVANCED_FACE('',(#3966,#3340),#28255,.T.);
#29295=ADVANCED_FACE('',(#3967),#1937,.F.);
#29296=ADVANCED_FACE('',(#3968),#487,.F.);
#29297=ADVANCED_FACE('',(#3969,#3341),#28256,.T.);
#29298=ADVANCED_FACE('',(#3970),#1938,.F.);
#29299=ADVANCED_FACE('',(#3971),#488,.F.);
#29300=ADVANCED_FACE('',(#3972,#3342),#28257,.T.);
#29301=ADVANCED_FACE('',(#3973),#1939,.F.);
#29302=ADVANCED_FACE('',(#3974),#489,.F.);
#29303=ADVANCED_FACE('',(#3975,#3343),#28258,.T.);
#29304=ADVANCED_FACE('',(#3976),#1940,.F.);
#29305=ADVANCED_FACE('',(#3977),#490,.F.);
#29306=ADVANCED_FACE('',(#3978,#3344),#28259,.T.);
#29307=ADVANCED_FACE('',(#3979),#1941,.F.);
#29308=ADVANCED_FACE('',(#3980),#491,.F.);
#29309=ADVANCED_FACE('',(#3981,#3345),#28260,.F.);
#29310=ADVANCED_FACE('',(#3982),#28261,.T.);
#29311=ADVANCED_FACE('',(#3983),#28262,.T.);
#29312=ADVANCED_FACE('',(#3984),#28263,.T.);
#29313=ADVANCED_FACE('',(#3985),#28264,.T.);
#29314=ADVANCED_FACE('',(#3986),#1942,.F.);
#29315=ADVANCED_FACE('',(#3987),#492,.F.);
#29316=ADVANCED_FACE('',(#3988,#3346),#28265,.T.);
#29317=ADVANCED_FACE('',(#3989),#1943,.F.);
#29318=ADVANCED_FACE('',(#3990),#493,.F.);
#29319=ADVANCED_FACE('',(#3991,#3347),#28266,.T.);
#29320=ADVANCED_FACE('',(#3992),#28267,.T.);
#29321=ADVANCED_FACE('',(#3993),#28268,.T.);
#29322=ADVANCED_FACE('',(#3994),#28269,.T.);
#29323=ADVANCED_FACE('',(#3995),#28270,.T.);
#29324=ADVANCED_FACE('',(#3996),#28271,.T.);
#29325=ADVANCED_FACE('',(#3997),#28272,.T.);
#29326=ADVANCED_FACE('',(#3998),#1944,.F.);
#29327=ADVANCED_FACE('',(#3999),#494,.F.);
#29328=ADVANCED_FACE('',(#4000,#3348),#28273,.T.);
#29329=ADVANCED_FACE('',(#4001),#1945,.F.);
#29330=ADVANCED_FACE('',(#4002),#495,.F.);
#29331=ADVANCED_FACE('',(#4003,#3349),#28274,.T.);
#29332=ADVANCED_FACE('',(#4004),#1946,.F.);
#29333=ADVANCED_FACE('',(#4005,#3350,#3351,#3352,#3353,#3354,#3355,#3356,
#3357,#3358,#3359,#3360,#3361,#3362,#3363,#3364,#3365,#3366,#3367,#3368,
#3369,#3370,#3371,#3372,#3373,#3374,#3375,#3376,#3377,#3378,#3379,#3380,
#3381,#3382,#3383,#3384,#3385,#3386,#3387,#3388,#3389,#3390,#3391),#28275,
 .F.);
#29334=ADVANCED_FACE('',(#4006),#1947,.F.);
#29335=ADVANCED_FACE('',(#4007),#1948,.F.);
#29336=ADVANCED_FACE('',(#4008),#1949,.F.);
#29337=ADVANCED_FACE('',(#4009),#1950,.F.);
#29338=ADVANCED_FACE('',(#4010),#1951,.F.);
#29339=ADVANCED_FACE('',(#4011),#1952,.F.);
#29340=ADVANCED_FACE('',(#4012),#1953,.F.);
#29341=ADVANCED_FACE('',(#4013),#1954,.F.);
#29342=ADVANCED_FACE('',(#4014),#496,.F.);
#29343=ADVANCED_FACE('',(#4015),#1955,.F.);
#29344=ADVANCED_FACE('',(#4016),#497,.F.);
#29345=ADVANCED_FACE('',(#4017),#1956,.F.);
#29346=ADVANCED_FACE('',(#4018),#1957,.F.);
#29347=ADVANCED_FACE('',(#4019),#28276,.T.);
#29348=ADVANCED_FACE('',(#4020),#28277,.T.);
#29349=ADVANCED_FACE('',(#4021),#28278,.T.);
#29350=ADVANCED_FACE('',(#4022),#1958,.F.);
#29351=ADVANCED_FACE('',(#4023),#498,.F.);
#29352=ADVANCED_FACE('',(#4024),#1959,.F.);
#29353=ADVANCED_FACE('',(#4025),#499,.F.);
#29354=ADVANCED_FACE('',(#4026),#1960,.F.);
#29355=ADVANCED_FACE('',(#4027),#500,.F.);
#29356=ADVANCED_FACE('',(#4028),#1961,.F.);
#29357=ADVANCED_FACE('',(#4029),#501,.F.);
#29358=ADVANCED_FACE('',(#4030),#1962,.F.);
#29359=ADVANCED_FACE('',(#4031),#502,.F.);
#29360=ADVANCED_FACE('',(#4032),#1963,.F.);
#29361=ADVANCED_FACE('',(#4033),#503,.F.);
#29362=ADVANCED_FACE('',(#4034),#1964,.F.);
#29363=ADVANCED_FACE('',(#4035),#504,.F.);
#29364=ADVANCED_FACE('',(#4036),#1965,.F.);
#29365=ADVANCED_FACE('',(#4037),#505,.F.);
#29366=ADVANCED_FACE('',(#4038),#1966,.F.);
#29367=ADVANCED_FACE('',(#4039),#506,.F.);
#29368=ADVANCED_FACE('',(#4040),#1967,.F.);
#29369=ADVANCED_FACE('',(#4041),#507,.F.);
#29370=ADVANCED_FACE('',(#4042),#1968,.F.);
#29371=ADVANCED_FACE('',(#4043),#508,.F.);
#29372=ADVANCED_FACE('',(#4044),#1969,.F.);
#29373=ADVANCED_FACE('',(#4045),#509,.F.);
#29374=ADVANCED_FACE('',(#4046),#1970,.F.);
#29375=ADVANCED_FACE('',(#4047),#1971,.F.);
#29376=ADVANCED_FACE('',(#4048),#1972,.F.);
#29377=ADVANCED_FACE('',(#4049),#510,.F.);
#29378=ADVANCED_FACE('',(#4050),#1973,.F.);
#29379=ADVANCED_FACE('',(#4051),#511,.F.);
#29380=ADVANCED_FACE('',(#4052),#1974,.F.);
#29381=ADVANCED_FACE('',(#4053),#512,.F.);
#29382=ADVANCED_FACE('',(#4054),#1975,.F.);
#29383=ADVANCED_FACE('',(#4055),#513,.F.);
#29384=ADVANCED_FACE('',(#4056),#1976,.F.);
#29385=ADVANCED_FACE('',(#4057),#514,.F.);
#29386=ADVANCED_FACE('',(#4058),#1977,.F.);
#29387=ADVANCED_FACE('',(#4059),#515,.F.);
#29388=ADVANCED_FACE('',(#4060),#1978,.F.);
#29389=ADVANCED_FACE('',(#4061),#516,.F.);
#29390=ADVANCED_FACE('',(#4062),#1979,.F.);
#29391=ADVANCED_FACE('',(#4063),#517,.F.);
#29392=ADVANCED_FACE('',(#4064),#1980,.F.);
#29393=ADVANCED_FACE('',(#4065),#518,.F.);
#29394=ADVANCED_FACE('',(#4066),#1981,.F.);
#29395=ADVANCED_FACE('',(#4067),#519,.F.);
#29396=ADVANCED_FACE('',(#4068),#1982,.F.);
#29397=ADVANCED_FACE('',(#4069),#520,.F.);
#29398=ADVANCED_FACE('',(#4070),#1983,.F.);
#29399=ADVANCED_FACE('',(#4071),#521,.F.);
#29400=ADVANCED_FACE('',(#4072),#1984,.F.);
#29401=ADVANCED_FACE('',(#4073),#522,.F.);
#29402=ADVANCED_FACE('',(#4074),#1985,.F.);
#29403=ADVANCED_FACE('',(#4075),#523,.F.);
#29404=ADVANCED_FACE('',(#4076),#1986,.F.);
#29405=ADVANCED_FACE('',(#4077),#524,.F.);
#29406=ADVANCED_FACE('',(#4078),#28279,.T.);
#29407=ADVANCED_FACE('',(#4079),#28280,.T.);
#29408=ADVANCED_FACE('',(#4080,#3392,#3393,#3394,#3395,#3396,#3397,#3398,
#3399,#3400,#3401,#3402,#3403,#3404,#3405,#3406,#3407,#3408,#3409,#3410,
#3411,#3412,#3413,#3414,#3415,#3416,#3417,#3418,#3419,#3420,#3421,#3422,
#3423,#3424,#3425,#3426,#3427,#3428,#3429,#3430,#3431,#3432,#3433),#28281,
 .T.);
#29409=ADVANCED_FACE('',(#4081),#1987,.F.);
#29410=ADVANCED_FACE('',(#4082),#1988,.F.);
#29411=ADVANCED_FACE('',(#4083),#1989,.F.);
#29412=ADVANCED_FACE('',(#4084),#1990,.F.);
#29413=ADVANCED_FACE('',(#4085),#1991,.F.);
#29414=ADVANCED_FACE('',(#4086),#1992,.F.);
#29415=ADVANCED_FACE('',(#4087),#1993,.F.);
#29416=ADVANCED_FACE('',(#4088),#1994,.F.);
#29417=ADVANCED_FACE('',(#4089),#1995,.F.);
#29418=ADVANCED_FACE('',(#4090),#525,.F.);
#29419=ADVANCED_FACE('',(#4091),#1996,.F.);
#29420=ADVANCED_FACE('',(#4092),#526,.F.);
#29421=ADVANCED_FACE('',(#4093),#1997,.F.);
#29422=ADVANCED_FACE('',(#4094),#527,.F.);
#29423=ADVANCED_FACE('',(#4095),#1998,.F.);
#29424=ADVANCED_FACE('',(#4096),#528,.F.);
#29425=ADVANCED_FACE('',(#4097),#1999,.F.);
#29426=ADVANCED_FACE('',(#4098),#529,.F.);
#29427=ADVANCED_FACE('',(#4099),#2000,.F.);
#29428=ADVANCED_FACE('',(#4100),#530,.F.);
#29429=ADVANCED_FACE('',(#4101),#2001,.F.);
#29430=ADVANCED_FACE('',(#4102),#531,.F.);
#29431=ADVANCED_FACE('',(#4103),#2002,.F.);
#29432=ADVANCED_FACE('',(#4104),#532,.F.);
#29433=ADVANCED_FACE('',(#4105),#2003,.F.);
#29434=ADVANCED_FACE('',(#4106),#533,.F.);
#29435=ADVANCED_FACE('',(#4107),#2004,.F.);
#29436=ADVANCED_FACE('',(#4108),#534,.F.);
#29437=ADVANCED_FACE('',(#4109),#2005,.F.);
#29438=ADVANCED_FACE('',(#4110),#2006,.F.);
#29439=ADVANCED_FACE('',(#4111),#2007,.F.);
#29440=ADVANCED_FACE('',(#4112),#2008,.F.);
#29441=ADVANCED_FACE('',(#4113),#2009,.F.);
#29442=ADVANCED_FACE('',(#4114),#2010,.F.);
#29443=ADVANCED_FACE('',(#4115),#2011,.F.);
#29444=ADVANCED_FACE('',(#4116),#2012,.F.);
#29445=ADVANCED_FACE('',(#4117),#2013,.F.);
#29446=ADVANCED_FACE('',(#4118),#2014,.F.);
#29447=ADVANCED_FACE('',(#4119),#2015,.F.);
#29448=ADVANCED_FACE('',(#4120),#2016,.F.);
#29449=ADVANCED_FACE('',(#4121),#2017,.F.);
#29450=ADVANCED_FACE('',(#4122),#2018,.F.);
#29451=ADVANCED_FACE('',(#4123),#2019,.F.);
#29452=ADVANCED_FACE('',(#4124),#2020,.F.);
#29453=ADVANCED_FACE('',(#4125),#2021,.F.);
#29454=ADVANCED_FACE('',(#4126),#2022,.F.);
#29455=ADVANCED_FACE('',(#4127),#2023,.F.);
#29456=ADVANCED_FACE('',(#4128),#2024,.F.);
#29457=ADVANCED_FACE('',(#4129),#2025,.F.);
#29458=ADVANCED_FACE('',(#4130),#2026,.F.);
#29459=ADVANCED_FACE('',(#4131),#2027,.F.);
#29460=ADVANCED_FACE('',(#4132),#535,.F.);
#29461=ADVANCED_FACE('',(#4133),#2028,.F.);
#29462=ADVANCED_FACE('',(#4134),#536,.F.);
#29463=ADVANCED_FACE('',(#4135),#537,.F.);
#29464=ADVANCED_FACE('',(#4136),#28282,.T.);
#30663=CLOSED_SHELL('',(#29283,#29284,#29285,#29286,#29287,#29288,#29289,
#29290,#29291,#29292,#29293,#29294,#29295,#29296,#29297,#29298,#29299,#29300,
#29301,#29302,#29303,#29304,#29305,#29306,#29307,#29308,#29309,#29310,#29311,
#29312,#29313,#29314,#29315,#29316,#29317,#29318,#29319,#29320,#29321,#29322,
#29323,#29324,#29325,#29326,#29327,#29328,#29329,#29330,#29331,#29332,#29333,
#29334,#29335,#29336,#29337,#29338,#29339,#29340,#29341,#29342,#29343,#29344,
#29345,#29346,#29347,#29348,#29349,#29350,#29351,#29352,#29353,#29354,#29355,
#29356,#29357,#29358,#29359,#29360,#29361,#29362,#29363,#29364,#29365,#29366,
#29367,#29368,#29369,#29370,#29371,#29372,#29373,#29374,#29375,#29376,#29377,
#29378,#29379,#29380,#29381,#29382,#29383,#29384,#29385,#29386,#29387,#29388,
#29389,#29390,#29391,#29392,#29393,#29394,#29395,#29396,#29397,#29398,#29399,
#29400,#29401,#29402,#29403,#29404,#29405,#29406,#29407,#29408,#29409,#29410,
#29411,#29412,#29413,#29414,#29415,#29416,#29417,#29418,#29419,#29420,#29421,
#29422,#29423,#29424,#29425,#29426,#29427,#29428,#29429,#29430,#29431,#29432,
#29433,#29434,#29435,#29436,#29437,#29438,#29439,#29440,#29441,#29442,#29443,
#29444,#29445,#29446,#29447,#29448,#29449,#29450,#29451,#29452,#29453,#29454,
#29455,#29456,#29457,#29458,#29459,#29460,#29461,#29462,#29463,#29464));
#31321=AXIS2_PLACEMENT_3D('',#43740,#34806,#34807);
#31322=AXIS2_PLACEMENT_3D('',#43741,#34808,#34809);
#31323=AXIS2_PLACEMENT_3D('',#43743,#34810,#34811);
#31324=AXIS2_PLACEMENT_3D('',#43746,#34813,#34814);
#31325=AXIS2_PLACEMENT_3D('',#43747,#34815,#34816);
#31326=AXIS2_PLACEMENT_3D('',#43750,#34818,#34819);
#31327=AXIS2_PLACEMENT_3D('',#43751,#34820,#34821);
#31328=AXIS2_PLACEMENT_3D('',#43753,#34822,#34823);
#31329=AXIS2_PLACEMENT_3D('',#43754,#34824,#34825);
#31330=AXIS2_PLACEMENT_3D('',#43756,#34826,#34827);
#31331=AXIS2_PLACEMENT_3D('',#43759,#34829,#34830);
#31332=AXIS2_PLACEMENT_3D('',#43760,#34831,#34832);
#31333=AXIS2_PLACEMENT_3D('',#43763,#34834,#34835);
#31334=AXIS2_PLACEMENT_3D('',#43764,#34836,#34837);
#31335=AXIS2_PLACEMENT_3D('',#43766,#34838,#34839);
#31336=AXIS2_PLACEMENT_3D('',#43767,#34840,#34841);
#31337=AXIS2_PLACEMENT_3D('',#43769,#34842,#34843);
#31338=AXIS2_PLACEMENT_3D('',#43772,#34845,#34846);
#31339=AXIS2_PLACEMENT_3D('',#43773,#34847,#34848);
#31340=AXIS2_PLACEMENT_3D('',#43776,#34850,#34851);
#31341=AXIS2_PLACEMENT_3D('',#43777,#34852,#34853);
#31342=AXIS2_PLACEMENT_3D('',#43779,#34854,#34855);
#31343=AXIS2_PLACEMENT_3D('',#43780,#34856,#34857);
#31344=AXIS2_PLACEMENT_3D('',#43782,#34858,#34859);
#31345=AXIS2_PLACEMENT_3D('',#43785,#34861,#34862);
#31346=AXIS2_PLACEMENT_3D('',#43786,#34863,#34864);
#31347=AXIS2_PLACEMENT_3D('',#43789,#34866,#34867);
#31348=AXIS2_PLACEMENT_3D('',#43790,#34868,#34869);
#31349=AXIS2_PLACEMENT_3D('',#43792,#34870,#34871);
#31350=AXIS2_PLACEMENT_3D('',#43793,#34872,#34873);
#31351=AXIS2_PLACEMENT_3D('',#43795,#34874,#34875);
#31352=AXIS2_PLACEMENT_3D('',#43798,#34877,#34878);
#31353=AXIS2_PLACEMENT_3D('',#43799,#34879,#34880);
#31354=AXIS2_PLACEMENT_3D('',#43802,#34882,#34883);
#31355=AXIS2_PLACEMENT_3D('',#43803,#34884,#34885);
#31356=AXIS2_PLACEMENT_3D('',#43805,#34886,#34887);
#31357=AXIS2_PLACEMENT_3D('',#43806,#34888,#34889);
#31358=AXIS2_PLACEMENT_3D('',#43808,#34890,#34891);
#31359=AXIS2_PLACEMENT_3D('',#43811,#34893,#34894);
#31360=AXIS2_PLACEMENT_3D('',#43812,#34895,#34896);
#31361=AXIS2_PLACEMENT_3D('',#43815,#34898,#34899);
#31362=AXIS2_PLACEMENT_3D('',#43816,#34900,#34901);
#31363=AXIS2_PLACEMENT_3D('',#43818,#34902,#34903);
#31364=AXIS2_PLACEMENT_3D('',#43819,#34904,#34905);
#31365=AXIS2_PLACEMENT_3D('',#43821,#34906,#34907);
#31366=AXIS2_PLACEMENT_3D('',#43824,#34909,#34910);
#31367=AXIS2_PLACEMENT_3D('',#43825,#34911,#34912);
#31368=AXIS2_PLACEMENT_3D('',#43828,#34914,#34915);
#31369=AXIS2_PLACEMENT_3D('',#43829,#34916,#34917);
#31370=AXIS2_PLACEMENT_3D('',#43831,#34918,#34919);
#31371=AXIS2_PLACEMENT_3D('',#43832,#34920,#34921);
#31372=AXIS2_PLACEMENT_3D('',#43834,#34922,#34923);
#31373=AXIS2_PLACEMENT_3D('',#43837,#34925,#34926);
#31374=AXIS2_PLACEMENT_3D('',#43838,#34927,#34928);
#31375=AXIS2_PLACEMENT_3D('',#43841,#34930,#34931);
#31376=AXIS2_PLACEMENT_3D('',#43842,#34932,#34933);
#31377=AXIS2_PLACEMENT_3D('',#43844,#34934,#34935);
#31378=AXIS2_PLACEMENT_3D('',#43845,#34936,#34937);
#31379=AXIS2_PLACEMENT_3D('',#43847,#34938,#34939);
#31380=AXIS2_PLACEMENT_3D('',#43850,#34941,#34942);
#31381=AXIS2_PLACEMENT_3D('',#43851,#34943,#34944);
#31382=AXIS2_PLACEMENT_3D('',#43853,#34945,#34946);
#31383=AXIS2_PLACEMENT_3D('',#43855,#34948,#34949);
#31384=AXIS2_PLACEMENT_3D('',#43857,#34950,#34951);
#31385=AXIS2_PLACEMENT_3D('',#43858,#34952,#34953);
#31386=AXIS2_PLACEMENT_3D('',#43871,#34960,#34961);
#31387=AXIS2_PLACEMENT_3D('',#43881,#34967,#34968);
#31388=AXIS2_PLACEMENT_3D('',#43885,#34971,#34972);
#31389=AXIS2_PLACEMENT_3D('',#43893,#34977,#34978);
#31390=AXIS2_PLACEMENT_3D('',#43895,#34979,#34980);
#31391=AXIS2_PLACEMENT_3D('',#43898,#34982,#34983);
#31392=AXIS2_PLACEMENT_3D('',#43899,#34984,#34985);
#31393=AXIS2_PLACEMENT_3D('',#43902,#34987,#34988);
#31394=AXIS2_PLACEMENT_3D('',#43903,#34989,#34990);
#31395=AXIS2_PLACEMENT_3D('',#43905,#34991,#34992);
#31396=AXIS2_PLACEMENT_3D('',#43906,#34993,#34994);
#31397=AXIS2_PLACEMENT_3D('',#43908,#34995,#34996);
#31398=AXIS2_PLACEMENT_3D('',#43911,#34998,#34999);
#31399=AXIS2_PLACEMENT_3D('',#43912,#35000,#35001);
#31400=AXIS2_PLACEMENT_3D('',#43915,#35003,#35004);
#31401=AXIS2_PLACEMENT_3D('',#43916,#35005,#35006);
#31402=AXIS2_PLACEMENT_3D('',#43918,#35007,#35008);
#31403=AXIS2_PLACEMENT_3D('',#43919,#35009,#35010);
#31404=AXIS2_PLACEMENT_3D('',#43932,#35017,#35018);
#31405=AXIS2_PLACEMENT_3D('',#43942,#35024,#35025);
#31406=AXIS2_PLACEMENT_3D('',#43946,#35028,#35029);
#31407=AXIS2_PLACEMENT_3D('',#43954,#35034,#35035);
#31408=AXIS2_PLACEMENT_3D('',#43960,#35039,#35040);
#31409=AXIS2_PLACEMENT_3D('',#43966,#35044,#35045);
#31410=AXIS2_PLACEMENT_3D('',#43968,#35046,#35047);
#31411=AXIS2_PLACEMENT_3D('',#43971,#35049,#35050);
#31412=AXIS2_PLACEMENT_3D('',#43972,#35051,#35052);
#31413=AXIS2_PLACEMENT_3D('',#43975,#35054,#35055);
#31414=AXIS2_PLACEMENT_3D('',#43976,#35056,#35057);
#31415=AXIS2_PLACEMENT_3D('',#43978,#35058,#35059);
#31416=AXIS2_PLACEMENT_3D('',#43979,#35060,#35061);
#31417=AXIS2_PLACEMENT_3D('',#43981,#35062,#35063);
#31418=AXIS2_PLACEMENT_3D('',#43984,#35065,#35066);
#31419=AXIS2_PLACEMENT_3D('',#43985,#35067,#35068);
#31420=AXIS2_PLACEMENT_3D('',#43988,#35070,#35071);
#31421=AXIS2_PLACEMENT_3D('',#43989,#35072,#35073);
#31422=AXIS2_PLACEMENT_3D('',#43991,#35074,#35075);
#31423=AXIS2_PLACEMENT_3D('',#43992,#35076,#35077);
#31424=AXIS2_PLACEMENT_3D('',#43994,#35078,#35079);
#31425=AXIS2_PLACEMENT_3D('',#43996,#35081,#35082);
#31426=AXIS2_PLACEMENT_3D('',#44000,#35085,#35086);
#31427=AXIS2_PLACEMENT_3D('',#44002,#35087,#35088);
#31428=AXIS2_PLACEMENT_3D('',#44004,#35089,#35090);
#31429=AXIS2_PLACEMENT_3D('',#44006,#35091,#35092);
#31430=AXIS2_PLACEMENT_3D('',#44008,#35093,#35094);
#31431=AXIS2_PLACEMENT_3D('',#44010,#35095,#35096);
#31432=AXIS2_PLACEMENT_3D('',#44012,#35097,#35098);
#31433=AXIS2_PLACEMENT_3D('',#44014,#35099,#35100);
#31434=AXIS2_PLACEMENT_3D('',#44016,#35101,#35102);
#31435=AXIS2_PLACEMENT_3D('',#44018,#35103,#35104);
#31436=AXIS2_PLACEMENT_3D('',#44020,#35105,#35106);
#31437=AXIS2_PLACEMENT_3D('',#44022,#35107,#35108);
#31438=AXIS2_PLACEMENT_3D('',#44024,#35109,#35110);
#31439=AXIS2_PLACEMENT_3D('',#44026,#35111,#35112);
#31440=AXIS2_PLACEMENT_3D('',#44028,#35113,#35114);
#31441=AXIS2_PLACEMENT_3D('',#44030,#35115,#35116);
#31442=AXIS2_PLACEMENT_3D('',#44032,#35117,#35118);
#31443=AXIS2_PLACEMENT_3D('',#44034,#35119,#35120);
#31444=AXIS2_PLACEMENT_3D('',#44036,#35121,#35122);
#31445=AXIS2_PLACEMENT_3D('',#44038,#35123,#35124);
#31446=AXIS2_PLACEMENT_3D('',#44040,#35125,#35126);
#31447=AXIS2_PLACEMENT_3D('',#44042,#35127,#35128);
#31448=AXIS2_PLACEMENT_3D('',#44044,#35129,#35130);
#31449=AXIS2_PLACEMENT_3D('',#44046,#35131,#35132);
#31450=AXIS2_PLACEMENT_3D('',#44048,#35133,#35134);
#31451=AXIS2_PLACEMENT_3D('',#44050,#35135,#35136);
#31452=AXIS2_PLACEMENT_3D('',#44052,#35137,#35138);
#31453=AXIS2_PLACEMENT_3D('',#44054,#35139,#35140);
#31454=AXIS2_PLACEMENT_3D('',#44056,#35141,#35142);
#31455=AXIS2_PLACEMENT_3D('',#44058,#35143,#35144);
#31456=AXIS2_PLACEMENT_3D('',#44060,#35145,#35146);
#31457=AXIS2_PLACEMENT_3D('',#44062,#35147,#35148);
#31458=AXIS2_PLACEMENT_3D('',#44064,#35149,#35150);
#31459=AXIS2_PLACEMENT_3D('',#44066,#35151,#35152);
#31460=AXIS2_PLACEMENT_3D('',#44068,#35153,#35154);
#31461=AXIS2_PLACEMENT_3D('',#44070,#35155,#35156);
#31462=AXIS2_PLACEMENT_3D('',#44072,#35157,#35158);
#31463=AXIS2_PLACEMENT_3D('',#44074,#35159,#35160);
#31464=AXIS2_PLACEMENT_3D('',#44076,#35161,#35162);
#31465=AXIS2_PLACEMENT_3D('',#44078,#35163,#35164);
#31466=AXIS2_PLACEMENT_3D('',#44080,#35165,#35166);
#31467=AXIS2_PLACEMENT_3D('',#44081,#35167,#35168);
#31468=AXIS2_PLACEMENT_3D('',#44083,#35170,#35171);
#31469=AXIS2_PLACEMENT_3D('',#44085,#35173,#35174);
#31470=AXIS2_PLACEMENT_3D('',#44087,#35176,#35177);
#31471=AXIS2_PLACEMENT_3D('',#44089,#35179,#35180);
#31472=AXIS2_PLACEMENT_3D('',#44091,#35182,#35183);
#31473=AXIS2_PLACEMENT_3D('',#44093,#35185,#35186);
#31474=AXIS2_PLACEMENT_3D('',#44095,#35188,#35189);
#31475=AXIS2_PLACEMENT_3D('',#44098,#35191,#35192);
#31476=AXIS2_PLACEMENT_3D('',#44099,#35193,#35194);
#31477=AXIS2_PLACEMENT_3D('',#44101,#35195,#35196);
#31478=AXIS2_PLACEMENT_3D('',#44103,#35198,#35199);
#31479=AXIS2_PLACEMENT_3D('',#44106,#35201,#35202);
#31480=AXIS2_PLACEMENT_3D('',#44107,#35203,#35204);
#31481=AXIS2_PLACEMENT_3D('',#44109,#35205,#35206);
#31482=AXIS2_PLACEMENT_3D('',#44111,#35208,#35209);
#31483=AXIS2_PLACEMENT_3D('',#44113,#35211,#35212);
#31484=AXIS2_PLACEMENT_3D('',#44115,#35214,#35215);
#31485=AXIS2_PLACEMENT_3D('',#44117,#35217,#35218);
#31486=AXIS2_PLACEMENT_3D('',#44119,#35220,#35221);
#31487=AXIS2_PLACEMENT_3D('',#44121,#35223,#35224);
#31488=AXIS2_PLACEMENT_3D('',#44124,#35226,#35227);
#31489=AXIS2_PLACEMENT_3D('',#44125,#35228,#35229);
#31490=AXIS2_PLACEMENT_3D('',#44127,#35230,#35231);
#31491=AXIS2_PLACEMENT_3D('',#44129,#35233,#35234);
#31492=AXIS2_PLACEMENT_3D('',#44132,#35236,#35237);
#31493=AXIS2_PLACEMENT_3D('',#44133,#35238,#35239);
#31494=AXIS2_PLACEMENT_3D('',#44135,#35240,#35241);
#31495=AXIS2_PLACEMENT_3D('',#44137,#35243,#35244);
#31496=AXIS2_PLACEMENT_3D('',#44140,#35246,#35247);
#31497=AXIS2_PLACEMENT_3D('',#44141,#35248,#35249);
#31498=AXIS2_PLACEMENT_3D('',#44143,#35250,#35251);
#31499=AXIS2_PLACEMENT_3D('',#44145,#35253,#35254);
#31500=AXIS2_PLACEMENT_3D('',#44148,#35256,#35257);
#31501=AXIS2_PLACEMENT_3D('',#44149,#35258,#35259);
#31502=AXIS2_PLACEMENT_3D('',#44151,#35260,#35261);
#31503=AXIS2_PLACEMENT_3D('',#44153,#35263,#35264);
#31504=AXIS2_PLACEMENT_3D('',#44156,#35266,#35267);
#31505=AXIS2_PLACEMENT_3D('',#44157,#35268,#35269);
#31506=AXIS2_PLACEMENT_3D('',#44159,#35270,#35271);
#31507=AXIS2_PLACEMENT_3D('',#44161,#35273,#35274);
#31508=AXIS2_PLACEMENT_3D('',#44164,#35276,#35277);
#31509=AXIS2_PLACEMENT_3D('',#44165,#35278,#35279);
#31510=AXIS2_PLACEMENT_3D('',#44167,#35280,#35281);
#31511=AXIS2_PLACEMENT_3D('',#44169,#35283,#35284);
#31512=AXIS2_PLACEMENT_3D('',#44172,#35286,#35287);
#31513=AXIS2_PLACEMENT_3D('',#44173,#35288,#35289);
#31514=AXIS2_PLACEMENT_3D('',#44175,#35290,#35291);
#31515=AXIS2_PLACEMENT_3D('',#44177,#35293,#35294);
#31516=AXIS2_PLACEMENT_3D('',#44180,#35296,#35297);
#31517=AXIS2_PLACEMENT_3D('',#44181,#35298,#35299);
#31518=AXIS2_PLACEMENT_3D('',#44183,#35300,#35301);
#31519=AXIS2_PLACEMENT_3D('',#44185,#35303,#35304);
#31520=AXIS2_PLACEMENT_3D('',#44188,#35306,#35307);
#31521=AXIS2_PLACEMENT_3D('',#44189,#35308,#35309);
#31522=AXIS2_PLACEMENT_3D('',#44191,#35310,#35311);
#31523=AXIS2_PLACEMENT_3D('',#44193,#35313,#35314);
#31524=AXIS2_PLACEMENT_3D('',#44196,#35316,#35317);
#31525=AXIS2_PLACEMENT_3D('',#44197,#35318,#35319);
#31526=AXIS2_PLACEMENT_3D('',#44199,#35320,#35321);
#31527=AXIS2_PLACEMENT_3D('',#44201,#35323,#35324);
#31528=AXIS2_PLACEMENT_3D('',#44204,#35326,#35327);
#31529=AXIS2_PLACEMENT_3D('',#44205,#35328,#35329);
#31530=AXIS2_PLACEMENT_3D('',#44207,#35330,#35331);
#31531=AXIS2_PLACEMENT_3D('',#44209,#35333,#35334);
#31532=AXIS2_PLACEMENT_3D('',#44212,#35336,#35337);
#31533=AXIS2_PLACEMENT_3D('',#44213,#35338,#35339);
#31534=AXIS2_PLACEMENT_3D('',#44215,#35340,#35341);
#31535=AXIS2_PLACEMENT_3D('',#44217,#35343,#35344);
#31536=AXIS2_PLACEMENT_3D('',#44219,#35346,#35347);
#31537=AXIS2_PLACEMENT_3D('',#44221,#35349,#35350);
#31538=AXIS2_PLACEMENT_3D('',#44224,#35352,#35353);
#31539=AXIS2_PLACEMENT_3D('',#44225,#35354,#35355);
#31540=AXIS2_PLACEMENT_3D('',#44227,#35356,#35357);
#31541=AXIS2_PLACEMENT_3D('',#44229,#35359,#35360);
#31542=AXIS2_PLACEMENT_3D('',#44232,#35362,#35363);
#31543=AXIS2_PLACEMENT_3D('',#44233,#35364,#35365);
#31544=AXIS2_PLACEMENT_3D('',#44235,#35366,#35367);
#31545=AXIS2_PLACEMENT_3D('',#44237,#35369,#35370);
#31546=AXIS2_PLACEMENT_3D('',#44240,#35372,#35373);
#31547=AXIS2_PLACEMENT_3D('',#44241,#35374,#35375);
#31548=AXIS2_PLACEMENT_3D('',#44243,#35376,#35377);
#31549=AXIS2_PLACEMENT_3D('',#44245,#35379,#35380);
#31550=AXIS2_PLACEMENT_3D('',#44248,#35382,#35383);
#31551=AXIS2_PLACEMENT_3D('',#44249,#35384,#35385);
#31552=AXIS2_PLACEMENT_3D('',#44251,#35386,#35387);
#31553=AXIS2_PLACEMENT_3D('',#44253,#35389,#35390);
#31554=AXIS2_PLACEMENT_3D('',#44256,#35392,#35393);
#31555=AXIS2_PLACEMENT_3D('',#44257,#35394,#35395);
#31556=AXIS2_PLACEMENT_3D('',#44259,#35396,#35397);
#31557=AXIS2_PLACEMENT_3D('',#44261,#35399,#35400);
#31558=AXIS2_PLACEMENT_3D('',#44264,#35402,#35403);
#31559=AXIS2_PLACEMENT_3D('',#44265,#35404,#35405);
#31560=AXIS2_PLACEMENT_3D('',#44267,#35406,#35407);
#31561=AXIS2_PLACEMENT_3D('',#44269,#35409,#35410);
#31562=AXIS2_PLACEMENT_3D('',#44272,#35412,#35413);
#31563=AXIS2_PLACEMENT_3D('',#44273,#35414,#35415);
#31564=AXIS2_PLACEMENT_3D('',#44275,#35416,#35417);
#31565=AXIS2_PLACEMENT_3D('',#44277,#35419,#35420);
#31566=AXIS2_PLACEMENT_3D('',#44280,#35422,#35423);
#31567=AXIS2_PLACEMENT_3D('',#44281,#35424,#35425);
#31568=AXIS2_PLACEMENT_3D('',#44283,#35426,#35427);
#31569=AXIS2_PLACEMENT_3D('',#44285,#35429,#35430);
#31570=AXIS2_PLACEMENT_3D('',#44288,#35432,#35433);
#31571=AXIS2_PLACEMENT_3D('',#44289,#35434,#35435);
#31572=AXIS2_PLACEMENT_3D('',#44291,#35436,#35437);
#31573=AXIS2_PLACEMENT_3D('',#44293,#35439,#35440);
#31574=AXIS2_PLACEMENT_3D('',#44296,#35442,#35443);
#31575=AXIS2_PLACEMENT_3D('',#44297,#35444,#35445);
#31576=AXIS2_PLACEMENT_3D('',#44299,#35446,#35447);
#31577=AXIS2_PLACEMENT_3D('',#44301,#35449,#35450);
#31578=AXIS2_PLACEMENT_3D('',#44304,#35452,#35453);
#31579=AXIS2_PLACEMENT_3D('',#44305,#35454,#35455);
#31580=AXIS2_PLACEMENT_3D('',#44307,#35456,#35457);
#31581=AXIS2_PLACEMENT_3D('',#44309,#35459,#35460);
#31582=AXIS2_PLACEMENT_3D('',#44312,#35462,#35463);
#31583=AXIS2_PLACEMENT_3D('',#44313,#35464,#35465);
#31584=AXIS2_PLACEMENT_3D('',#44315,#35466,#35467);
#31585=AXIS2_PLACEMENT_3D('',#44317,#35469,#35470);
#31586=AXIS2_PLACEMENT_3D('',#44320,#35472,#35473);
#31587=AXIS2_PLACEMENT_3D('',#44321,#35474,#35475);
#31588=AXIS2_PLACEMENT_3D('',#44323,#35476,#35477);
#31589=AXIS2_PLACEMENT_3D('',#44325,#35479,#35480);
#31590=AXIS2_PLACEMENT_3D('',#44328,#35482,#35483);
#31591=AXIS2_PLACEMENT_3D('',#44329,#35484,#35485);
#31592=AXIS2_PLACEMENT_3D('',#44331,#35486,#35487);
#31593=AXIS2_PLACEMENT_3D('',#44333,#35489,#35490);
#31594=AXIS2_PLACEMENT_3D('',#44336,#35492,#35493);
#31595=AXIS2_PLACEMENT_3D('',#44337,#35494,#35495);
#31596=AXIS2_PLACEMENT_3D('',#44339,#35496,#35497);
#31597=AXIS2_PLACEMENT_3D('',#44341,#35499,#35500);
#31598=AXIS2_PLACEMENT_3D('',#44344,#35503,#35504);
#31599=AXIS2_PLACEMENT_3D('',#44346,#35506,#35507);
#31600=AXIS2_PLACEMENT_3D('',#44348,#35508,#35509);
#31601=AXIS2_PLACEMENT_3D('',#44350,#35510,#35511);
#31602=AXIS2_PLACEMENT_3D('',#44352,#35512,#35513);
#31603=AXIS2_PLACEMENT_3D('',#44354,#35514,#35515);
#31604=AXIS2_PLACEMENT_3D('',#44356,#35516,#35517);
#31605=AXIS2_PLACEMENT_3D('',#44358,#35518,#35519);
#31606=AXIS2_PLACEMENT_3D('',#44360,#35520,#35521);
#31607=AXIS2_PLACEMENT_3D('',#44362,#35522,#35523);
#31608=AXIS2_PLACEMENT_3D('',#44364,#35524,#35525);
#31609=AXIS2_PLACEMENT_3D('',#44366,#35526,#35527);
#31610=AXIS2_PLACEMENT_3D('',#44368,#35528,#35529);
#31611=AXIS2_PLACEMENT_3D('',#44370,#35530,#35531);
#31612=AXIS2_PLACEMENT_3D('',#44372,#35532,#35533);
#31613=AXIS2_PLACEMENT_3D('',#44374,#35534,#35535);
#31614=AXIS2_PLACEMENT_3D('',#44376,#35536,#35537);
#31615=AXIS2_PLACEMENT_3D('',#44378,#35538,#35539);
#31616=AXIS2_PLACEMENT_3D('',#44380,#35540,#35541);
#31617=AXIS2_PLACEMENT_3D('',#44382,#35542,#35543);
#31618=AXIS2_PLACEMENT_3D('',#44384,#35544,#35545);
#31619=AXIS2_PLACEMENT_3D('',#44386,#35546,#35547);
#31620=AXIS2_PLACEMENT_3D('',#44388,#35548,#35549);
#31621=AXIS2_PLACEMENT_3D('',#44390,#35550,#35551);
#31622=AXIS2_PLACEMENT_3D('',#44392,#35552,#35553);
#31623=AXIS2_PLACEMENT_3D('',#44394,#35554,#35555);
#31624=AXIS2_PLACEMENT_3D('',#44396,#35556,#35557);
#31625=AXIS2_PLACEMENT_3D('',#44398,#35558,#35559);
#31626=AXIS2_PLACEMENT_3D('',#44400,#35560,#35561);
#31627=AXIS2_PLACEMENT_3D('',#44402,#35562,#35563);
#31628=AXIS2_PLACEMENT_3D('',#44404,#35564,#35565);
#31629=AXIS2_PLACEMENT_3D('',#44406,#35566,#35567);
#31630=AXIS2_PLACEMENT_3D('',#44408,#35568,#35569);
#31631=AXIS2_PLACEMENT_3D('',#44410,#35570,#35571);
#31632=AXIS2_PLACEMENT_3D('',#44412,#35572,#35573);
#31633=AXIS2_PLACEMENT_3D('',#44414,#35574,#35575);
#31634=AXIS2_PLACEMENT_3D('',#44416,#35576,#35577);
#31635=AXIS2_PLACEMENT_3D('',#44418,#35578,#35579);
#31636=AXIS2_PLACEMENT_3D('',#44420,#35580,#35581);
#31637=AXIS2_PLACEMENT_3D('',#44422,#35582,#35583);
#31638=AXIS2_PLACEMENT_3D('',#44424,#35584,#35585);
#31639=AXIS2_PLACEMENT_3D('',#44426,#35586,#35587);
#31640=AXIS2_PLACEMENT_3D('',#44428,#35588,#35589);
#31641=AXIS2_PLACEMENT_3D('',#44430,#35590,#35591);
#31642=AXIS2_PLACEMENT_3D('',#44431,#35592,#35593);
#31643=AXIS2_PLACEMENT_3D('',#44433,#35595,#35596);
#31644=AXIS2_PLACEMENT_3D('',#44435,#35598,#35599);
#31645=AXIS2_PLACEMENT_3D('',#44437,#35601,#35602);
#31646=AXIS2_PLACEMENT_3D('',#44439,#35604,#35605);
#31647=AXIS2_PLACEMENT_3D('',#44441,#35607,#35608);
#31648=AXIS2_PLACEMENT_3D('',#44443,#35610,#35611);
#31649=AXIS2_PLACEMENT_3D('',#44445,#35613,#35614);
#31650=AXIS2_PLACEMENT_3D('',#44447,#35616,#35617);
#31651=AXIS2_PLACEMENT_3D('',#44450,#35619,#35620);
#31652=AXIS2_PLACEMENT_3D('',#44451,#35621,#35622);
#31653=AXIS2_PLACEMENT_3D('',#44453,#35624,#35625);
#31654=AXIS2_PLACEMENT_3D('',#44456,#35627,#35628);
#31655=AXIS2_PLACEMENT_3D('',#44457,#35629,#35630);
#31656=AXIS2_PLACEMENT_3D('',#44459,#35632,#35633);
#31657=AXIS2_PLACEMENT_3D('',#44462,#35635,#35636);
#31658=AXIS2_PLACEMENT_3D('',#44463,#35637,#35638);
#31659=AXIS2_PLACEMENT_3D('',#44465,#35640,#35641);
#31660=AXIS2_PLACEMENT_3D('',#44468,#35643,#35644);
#31661=AXIS2_PLACEMENT_3D('',#44469,#35645,#35646);
#31662=AXIS2_PLACEMENT_3D('',#44471,#35648,#35649);
#31663=AXIS2_PLACEMENT_3D('',#44474,#35651,#35652);
#31664=AXIS2_PLACEMENT_3D('',#44475,#35653,#35654);
#31665=AXIS2_PLACEMENT_3D('',#44477,#35656,#35657);
#31666=AXIS2_PLACEMENT_3D('',#44480,#35659,#35660);
#31667=AXIS2_PLACEMENT_3D('',#44481,#35661,#35662);
#31668=AXIS2_PLACEMENT_3D('',#44483,#35664,#35665);
#31669=AXIS2_PLACEMENT_3D('',#44486,#35667,#35668);
#31670=AXIS2_PLACEMENT_3D('',#44487,#35669,#35670);
#31671=AXIS2_PLACEMENT_3D('',#44489,#35672,#35673);
#31672=AXIS2_PLACEMENT_3D('',#44492,#35675,#35676);
#31673=AXIS2_PLACEMENT_3D('',#44493,#35677,#35678);
#31674=AXIS2_PLACEMENT_3D('',#44495,#35680,#35681);
#31675=AXIS2_PLACEMENT_3D('',#44498,#35683,#35684);
#31676=AXIS2_PLACEMENT_3D('',#44499,#35685,#35686);
#31677=AXIS2_PLACEMENT_3D('',#44501,#35688,#35689);
#31678=AXIS2_PLACEMENT_3D('',#44504,#35691,#35692);
#31679=AXIS2_PLACEMENT_3D('',#44505,#35693,#35694);
#31680=AXIS2_PLACEMENT_3D('',#44507,#35696,#35697);
#31681=AXIS2_PLACEMENT_3D('',#44509,#35699,#35700);
#31682=AXIS2_PLACEMENT_3D('',#44511,#35702,#35703);
#31683=AXIS2_PLACEMENT_3D('',#44513,#35705,#35706);
#31684=AXIS2_PLACEMENT_3D('',#44515,#35708,#35709);
#31685=AXIS2_PLACEMENT_3D('',#44517,#35711,#35712);
#31686=AXIS2_PLACEMENT_3D('',#44519,#35714,#35715);
#31687=AXIS2_PLACEMENT_3D('',#44521,#35717,#35718);
#31688=AXIS2_PLACEMENT_3D('',#44523,#35720,#35721);
#31689=AXIS2_PLACEMENT_3D('',#44525,#35723,#35724);
#31690=AXIS2_PLACEMENT_3D('',#44527,#35726,#35727);
#31691=AXIS2_PLACEMENT_3D('',#44529,#35729,#35730);
#31692=AXIS2_PLACEMENT_3D('',#44531,#35732,#35733);
#31693=AXIS2_PLACEMENT_3D('',#44533,#35735,#35736);
#31694=AXIS2_PLACEMENT_3D('',#44535,#35738,#35739);
#31695=AXIS2_PLACEMENT_3D('',#44537,#35741,#35742);
#31696=AXIS2_PLACEMENT_3D('',#44539,#35744,#35745);
#31697=AXIS2_PLACEMENT_3D('',#44541,#35747,#35748);
#31698=AXIS2_PLACEMENT_3D('',#44543,#35750,#35751);
#31699=AXIS2_PLACEMENT_3D('',#44545,#35753,#35754);
#31700=AXIS2_PLACEMENT_3D('',#44547,#35756,#35757);
#31701=AXIS2_PLACEMENT_3D('',#44549,#35759,#35760);
#31702=AXIS2_PLACEMENT_3D('',#44551,#35762,#35763);
#31703=AXIS2_PLACEMENT_3D('',#44554,#35765,#35766);
#31704=AXIS2_PLACEMENT_3D('',#44555,#35767,#35768);
#31705=AXIS2_PLACEMENT_3D('',#44557,#35770,#35771);
#31706=AXIS2_PLACEMENT_3D('',#44560,#35773,#35774);
#31707=AXIS2_PLACEMENT_3D('',#44561,#35775,#35776);
#31708=AXIS2_PLACEMENT_3D('',#44563,#35778,#35779);
#31709=AXIS2_PLACEMENT_3D('',#44565,#35781,#35782);
#34806=DIRECTION('axis',(0.,0.,1.));
#34807=DIRECTION('refdir',(1.,0.,0.));
#34808=DIRECTION('center_axis',(0.,0.,1.));
#34809=DIRECTION('ref_axis',(1.,0.,0.));
#34810=DIRECTION('center_axis',(0.,0.,-1.));
#34811=DIRECTION('ref_axis',(1.,0.,0.));
#34812=DIRECTION('',(-0.707106781186547,8.65956056235493E-17,0.707106781186547));
#34813=DIRECTION('center_axis',(0.,0.,1.));
#34814=DIRECTION('ref_axis',(1.,0.,0.));
#34815=DIRECTION('center_axis',(0.,0.,-1.));
#34816=DIRECTION('ref_axis',(1.,0.,0.));
#34817=DIRECTION('',(0.,0.,-1.));
#34818=DIRECTION('center_axis',(0.,0.,1.));
#34819=DIRECTION('ref_axis',(1.,0.,0.));
#34820=DIRECTION('center_axis',(0.,0.,1.));
#34821=DIRECTION('ref_axis',(1.,0.,0.));
#34822=DIRECTION('center_axis',(0.,0.,-1.));
#34823=DIRECTION('ref_axis',(1.,0.,0.));
#34824=DIRECTION('center_axis',(0.,0.,1.));
#34825=DIRECTION('ref_axis',(1.,0.,0.));
#34826=DIRECTION('center_axis',(0.,0.,-1.));
#34827=DIRECTION('ref_axis',(1.,0.,0.));
#34828=DIRECTION('',(-0.707106781186547,8.65956056235493E-17,0.707106781186547));
#34829=DIRECTION('center_axis',(0.,0.,1.));
#34830=DIRECTION('ref_axis',(1.,0.,0.));
#34831=DIRECTION('center_axis',(0.,0.,-1.));
#34832=DIRECTION('ref_axis',(1.,0.,0.));
#34833=DIRECTION('',(0.,0.,-1.));
#34834=DIRECTION('center_axis',(0.,0.,1.));
#34835=DIRECTION('ref_axis',(1.,0.,0.));
#34836=DIRECTION('center_axis',(0.,0.,1.));
#34837=DIRECTION('ref_axis',(1.,0.,0.));
#34838=DIRECTION('center_axis',(0.,0.,-1.));
#34839=DIRECTION('ref_axis',(1.,0.,0.));
#34840=DIRECTION('center_axis',(0.,0.,1.));
#34841=DIRECTION('ref_axis',(1.,0.,0.));
#34842=DIRECTION('center_axis',(0.,0.,-1.));
#34843=DIRECTION('ref_axis',(1.,0.,0.));
#34844=DIRECTION('',(-0.707106781186549,8.65956056235495E-17,0.707106781186546));
#34845=DIRECTION('center_axis',(0.,0.,1.));
#34846=DIRECTION('ref_axis',(1.,0.,0.));
#34847=DIRECTION('center_axis',(0.,0.,-1.));
#34848=DIRECTION('ref_axis',(1.,0.,0.));
#34849=DIRECTION('',(0.,0.,-1.));
#34850=DIRECTION('center_axis',(0.,0.,1.));
#34851=DIRECTION('ref_axis',(1.,0.,0.));
#34852=DIRECTION('center_axis',(0.,0.,1.));
#34853=DIRECTION('ref_axis',(1.,0.,0.));
#34854=DIRECTION('center_axis',(0.,0.,-1.));
#34855=DIRECTION('ref_axis',(1.,0.,0.));
#34856=DIRECTION('center_axis',(0.,0.,1.));
#34857=DIRECTION('ref_axis',(1.,0.,0.));
#34858=DIRECTION('center_axis',(0.,0.,-1.));
#34859=DIRECTION('ref_axis',(1.,0.,0.));
#34860=DIRECTION('',(-0.707106781186549,8.65956056235495E-17,0.707106781186546));
#34861=DIRECTION('center_axis',(0.,0.,1.));
#34862=DIRECTION('ref_axis',(1.,0.,0.));
#34863=DIRECTION('center_axis',(0.,0.,-1.));
#34864=DIRECTION('ref_axis',(1.,0.,0.));
#34865=DIRECTION('',(0.,0.,-1.));
#34866=DIRECTION('center_axis',(0.,0.,1.));
#34867=DIRECTION('ref_axis',(1.,0.,0.));
#34868=DIRECTION('center_axis',(0.,0.,1.));
#34869=DIRECTION('ref_axis',(1.,0.,0.));
#34870=DIRECTION('center_axis',(0.,0.,-1.));
#34871=DIRECTION('ref_axis',(1.,0.,0.));
#34872=DIRECTION('center_axis',(0.,0.,1.));
#34873=DIRECTION('ref_axis',(1.,0.,0.));
#34874=DIRECTION('center_axis',(0.,0.,-1.));
#34875=DIRECTION('ref_axis',(1.,0.,0.));
#34876=DIRECTION('',(-0.707106781186549,8.65956056235495E-17,0.707106781186546));
#34877=DIRECTION('center_axis',(0.,0.,1.));
#34878=DIRECTION('ref_axis',(1.,0.,0.));
#34879=DIRECTION('center_axis',(0.,0.,-1.));
#34880=DIRECTION('ref_axis',(1.,0.,0.));
#34881=DIRECTION('',(0.,0.,-1.));
#34882=DIRECTION('center_axis',(0.,0.,1.));
#34883=DIRECTION('ref_axis',(1.,0.,0.));
#34884=DIRECTION('center_axis',(0.,0.,1.));
#34885=DIRECTION('ref_axis',(1.,0.,0.));
#34886=DIRECTION('center_axis',(0.,0.,-1.));
#34887=DIRECTION('ref_axis',(1.,0.,0.));
#34888=DIRECTION('center_axis',(0.,0.,1.));
#34889=DIRECTION('ref_axis',(1.,0.,0.));
#34890=DIRECTION('center_axis',(0.,0.,-1.));
#34891=DIRECTION('ref_axis',(1.,0.,0.));
#34892=DIRECTION('',(-0.707106781186547,8.65956056235493E-17,0.707106781186547));
#34893=DIRECTION('center_axis',(0.,0.,1.));
#34894=DIRECTION('ref_axis',(1.,0.,0.));
#34895=DIRECTION('center_axis',(0.,0.,-1.));
#34896=DIRECTION('ref_axis',(1.,0.,0.));
#34897=DIRECTION('',(0.,0.,-1.));
#34898=DIRECTION('center_axis',(0.,0.,1.));
#34899=DIRECTION('ref_axis',(1.,0.,0.));
#34900=DIRECTION('center_axis',(0.,0.,1.));
#34901=DIRECTION('ref_axis',(1.,0.,0.));
#34902=DIRECTION('center_axis',(0.,0.,-1.));
#34903=DIRECTION('ref_axis',(1.,0.,0.));
#34904=DIRECTION('center_axis',(0.,0.,1.));
#34905=DIRECTION('ref_axis',(1.,0.,0.));
#34906=DIRECTION('center_axis',(0.,0.,-1.));
#34907=DIRECTION('ref_axis',(1.,0.,0.));
#34908=DIRECTION('',(-0.707106781186547,8.65956056235493E-17,0.707106781186547));
#34909=DIRECTION('center_axis',(0.,0.,1.));
#34910=DIRECTION('ref_axis',(1.,0.,0.));
#34911=DIRECTION('center_axis',(0.,0.,-1.));
#34912=DIRECTION('ref_axis',(1.,0.,0.));
#34913=DIRECTION('',(0.,0.,-1.));
#34914=DIRECTION('center_axis',(0.,0.,1.));
#34915=DIRECTION('ref_axis',(1.,0.,0.));
#34916=DIRECTION('center_axis',(0.,0.,1.));
#34917=DIRECTION('ref_axis',(1.,0.,0.));
#34918=DIRECTION('center_axis',(0.,0.,-1.));
#34919=DIRECTION('ref_axis',(1.,0.,0.));
#34920=DIRECTION('center_axis',(0.,0.,1.));
#34921=DIRECTION('ref_axis',(1.,0.,0.));
#34922=DIRECTION('center_axis',(0.,0.,-1.));
#34923=DIRECTION('ref_axis',(1.,0.,0.));
#34924=DIRECTION('',(-0.707106781186547,8.65956056235493E-17,0.707106781186547));
#34925=DIRECTION('center_axis',(0.,0.,1.));
#34926=DIRECTION('ref_axis',(1.,0.,0.));
#34927=DIRECTION('center_axis',(0.,0.,-1.));
#34928=DIRECTION('ref_axis',(1.,0.,0.));
#34929=DIRECTION('',(0.,0.,-1.));
#34930=DIRECTION('center_axis',(0.,0.,1.));
#34931=DIRECTION('ref_axis',(1.,0.,0.));
#34932=DIRECTION('center_axis',(0.,0.,1.));
#34933=DIRECTION('ref_axis',(1.,0.,0.));
#34934=DIRECTION('center_axis',(0.,0.,-1.));
#34935=DIRECTION('ref_axis',(1.,0.,0.));
#34936=DIRECTION('center_axis',(0.,0.,-1.));
#34937=DIRECTION('ref_axis',(1.,0.,0.));
#34938=DIRECTION('center_axis',(0.,0.,1.));
#34939=DIRECTION('ref_axis',(1.,0.,0.));
#34940=DIRECTION('',(-0.707106781186547,-8.65956056235493E-17,-0.707106781186547));
#34941=DIRECTION('center_axis',(0.,0.,-1.));
#34942=DIRECTION('ref_axis',(1.,0.,0.));
#34943=DIRECTION('center_axis',(0.,0.,-1.));
#34944=DIRECTION('ref_axis',(1.,0.,0.));
#34945=DIRECTION('center_axis',(0.,0.,-1.));
#34946=DIRECTION('ref_axis',(1.,0.,0.));
#34947=DIRECTION('',(0.,0.,-1.));
#34948=DIRECTION('center_axis',(0.,0.,1.));
#34949=DIRECTION('ref_axis',(1.,0.,0.));
#34950=DIRECTION('center_axis',(0.,0.,1.));
#34951=DIRECTION('ref_axis',(1.,0.,0.));
#34952=DIRECTION('center_axis',(0.707106781186548,-0.707106781186548,0.));
#34953=DIRECTION('ref_axis',(0.,0.,-1.));
#34954=DIRECTION('',(-0.577350269189629,-0.577350269189629,-0.577350269189619));
#34955=DIRECTION('',(0.,0.,-1.));
#34956=DIRECTION('',(0.577350269189629,0.577350269189629,-0.577350269189619));
#34957=DIRECTION('',(0.577350269189629,0.577350269189629,0.577350269189619));
#34958=DIRECTION('',(0.,0.,1.));
#34959=DIRECTION('',(-0.577350269189629,-0.577350269189629,0.577350269189619));
#34960=DIRECTION('center_axis',(0.707106781186541,0.,0.707106781186554));
#34961=DIRECTION('ref_axis',(0.707106781186554,0.,-0.707106781186541));
#34962=DIRECTION('',(0.,1.,0.));
#34963=DIRECTION('',(0.577350269189629,-0.577350269189629,-0.577350269189619));
#34964=DIRECTION('',(0.577350269189636,0.577350269189616,-0.577350269189626));
#34965=DIRECTION('',(0.,-1.,0.));
#34966=DIRECTION('',(0.577350269189616,-0.577350269189636,-0.577350269189626));
#34967=DIRECTION('center_axis',(1.,0.,0.));
#34968=DIRECTION('ref_axis',(0.,1.,0.));
#34969=DIRECTION('',(0.,-1.,0.));
#34970=DIRECTION('',(0.,0.,-1.));
#34971=DIRECTION('center_axis',(0.707106781186541,0.,-0.707106781186554));
#34972=DIRECTION('ref_axis',(-0.707106781186554,0.,-0.707106781186541));
#34973=DIRECTION('',(0.577350269189629,-0.577350269189629,0.577350269189619));
#34974=DIRECTION('',(0.,1.,0.));
#34975=DIRECTION('',(0.577350269189629,0.577350269189629,0.577350269189619));
#34976=DIRECTION('',(-0.577350269189629,0.577350269189629,-0.577350269189619));
#34977=DIRECTION('center_axis',(0.,0.,1.));
#34978=DIRECTION('ref_axis',(1.,0.,0.));
#34979=DIRECTION('center_axis',(0.,0.,-1.));
#34980=DIRECTION('ref_axis',(1.,0.,0.));
#34981=DIRECTION('',(-0.707106781186549,8.65956056235495E-17,0.707106781186546));
#34982=DIRECTION('center_axis',(0.,0.,1.));
#34983=DIRECTION('ref_axis',(1.,0.,0.));
#34984=DIRECTION('center_axis',(0.,0.,-1.));
#34985=DIRECTION('ref_axis',(1.,0.,0.));
#34986=DIRECTION('',(0.,0.,-1.));
#34987=DIRECTION('center_axis',(0.,0.,1.));
#34988=DIRECTION('ref_axis',(1.,0.,0.));
#34989=DIRECTION('center_axis',(0.,0.,1.));
#34990=DIRECTION('ref_axis',(1.,0.,0.));
#34991=DIRECTION('center_axis',(0.,0.,-1.));
#34992=DIRECTION('ref_axis',(1.,0.,0.));
#34993=DIRECTION('center_axis',(0.,0.,1.));
#34994=DIRECTION('ref_axis',(1.,0.,0.));
#34995=DIRECTION('center_axis',(0.,0.,-1.));
#34996=DIRECTION('ref_axis',(1.,0.,0.));
#34997=DIRECTION('',(-0.707106781186548,8.65956056235493E-17,0.707106781186548));
#34998=DIRECTION('center_axis',(0.,0.,1.));
#34999=DIRECTION('ref_axis',(1.,0.,0.));
#35000=DIRECTION('center_axis',(0.,0.,-1.));
#35001=DIRECTION('ref_axis',(1.,0.,0.));
#35002=DIRECTION('',(0.,0.,-1.));
#35003=DIRECTION('center_axis',(0.,0.,1.));
#35004=DIRECTION('ref_axis',(1.,0.,0.));
#35005=DIRECTION('center_axis',(0.,0.,1.));
#35006=DIRECTION('ref_axis',(1.,0.,0.));
#35007=DIRECTION('center_axis',(0.,0.,-1.));
#35008=DIRECTION('ref_axis',(1.,0.,0.));
#35009=DIRECTION('center_axis',(-0.707106781186548,-0.707106781186548,0.));
#35010=DIRECTION('ref_axis',(0.,0.,1.));
#35011=DIRECTION('',(-0.577350269189629,0.577350269189629,-0.577350269189619));
#35012=DIRECTION('',(0.,0.,-1.));
#35013=DIRECTION('',(0.577350269189629,-0.577350269189629,-0.577350269189619));
#35014=DIRECTION('',(0.577350269189629,-0.577350269189629,0.577350269189619));
#35015=DIRECTION('',(0.,0.,1.));
#35016=DIRECTION('',(-0.577350269189629,0.577350269189629,0.577350269189619));
#35017=DIRECTION('center_axis',(-0.707106781186541,0.,-0.707106781186554));
#35018=DIRECTION('ref_axis',(-0.707106781186554,0.,0.707106781186541));
#35019=DIRECTION('',(0.,1.,0.));
#35020=DIRECTION('',(-0.577350269189629,-0.577350269189629,0.577350269189619));
#35021=DIRECTION('',(0.577350269189616,-0.577350269189636,-0.577350269189626));
#35022=DIRECTION('',(0.,-1.,0.));
#35023=DIRECTION('',(-0.577350269189629,-0.577350269189629,0.577350269189619));
#35024=DIRECTION('center_axis',(-1.,0.,0.));
#35025=DIRECTION('ref_axis',(0.,-1.,0.));
#35026=DIRECTION('',(0.,-1.,0.));
#35027=DIRECTION('',(0.,0.,1.));
#35028=DIRECTION('center_axis',(-0.707106781186541,0.,0.707106781186554));
#35029=DIRECTION('ref_axis',(0.707106781186554,0.,0.707106781186541));
#35030=DIRECTION('',(-0.577350269189636,-0.577350269189616,-0.577350269189626));
#35031=DIRECTION('',(0.,1.,0.));
#35032=DIRECTION('',(-0.577350269189616,0.577350269189636,-0.577350269189626));
#35033=DIRECTION('',(0.577350269189629,0.577350269189629,0.577350269189619));
#35034=DIRECTION('center_axis',(0.707106781186548,0.707106781186548,0.));
#35035=DIRECTION('ref_axis',(0.,0.,-1.));
#35036=DIRECTION('',(-0.577350269189629,0.577350269189629,0.577350269189619));
#35037=DIRECTION('',(0.,0.,1.));
#35038=DIRECTION('',(0.577350269189629,-0.577350269189629,0.577350269189619));
#35039=DIRECTION('center_axis',(-0.707106781186548,0.707106781186548,0.));
#35040=DIRECTION('ref_axis',(0.,0.,1.));
#35041=DIRECTION('',(0.577350269189629,0.577350269189629,-0.577350269189619));
#35042=DIRECTION('',(0.,0.,-1.));
#35043=DIRECTION('',(-0.577350269189629,-0.577350269189629,-0.577350269189619));
#35044=DIRECTION('center_axis',(0.,0.,1.));
#35045=DIRECTION('ref_axis',(1.,0.,0.));
#35046=DIRECTION('center_axis',(0.,0.,-1.));
#35047=DIRECTION('ref_axis',(1.,0.,0.));
#35048=DIRECTION('',(-0.707106781186547,8.65956056235493E-17,0.707106781186547));
#35049=DIRECTION('center_axis',(0.,0.,1.));
#35050=DIRECTION('ref_axis',(1.,0.,0.));
#35051=DIRECTION('center_axis',(0.,0.,-1.));
#35052=DIRECTION('ref_axis',(1.,0.,0.));
#35053=DIRECTION('',(0.,0.,-1.));
#35054=DIRECTION('center_axis',(0.,0.,1.));
#35055=DIRECTION('ref_axis',(1.,0.,0.));
#35056=DIRECTION('center_axis',(0.,0.,1.));
#35057=DIRECTION('ref_axis',(1.,0.,0.));
#35058=DIRECTION('center_axis',(0.,0.,-1.));
#35059=DIRECTION('ref_axis',(1.,0.,0.));
#35060=DIRECTION('center_axis',(0.,0.,1.));
#35061=DIRECTION('ref_axis',(1.,0.,0.));
#35062=DIRECTION('center_axis',(0.,0.,-1.));
#35063=DIRECTION('ref_axis',(1.,0.,0.));
#35064=DIRECTION('',(-0.707106781186547,8.65956056235493E-17,0.707106781186547));
#35065=DIRECTION('center_axis',(0.,0.,1.));
#35066=DIRECTION('ref_axis',(1.,0.,0.));
#35067=DIRECTION('center_axis',(0.,0.,-1.));
#35068=DIRECTION('ref_axis',(1.,0.,0.));
#35069=DIRECTION('',(0.,0.,-1.));
#35070=DIRECTION('center_axis',(0.,0.,1.));
#35071=DIRECTION('ref_axis',(1.,0.,0.));
#35072=DIRECTION('center_axis',(0.,0.,1.));
#35073=DIRECTION('ref_axis',(1.,0.,0.));
#35074=DIRECTION('center_axis',(0.,0.,-1.));
#35075=DIRECTION('ref_axis',(1.,0.,0.));
#35076=DIRECTION('center_axis',(0.,0.,-1.));
#35077=DIRECTION('ref_axis',(1.,0.,0.));
#35078=DIRECTION('center_axis',(0.,0.,-1.));
#35079=DIRECTION('ref_axis',(1.,0.,0.));
#35080=DIRECTION('',(0.707106781186547,-8.65956056235493E-17,0.707106781186547));
#35081=DIRECTION('center_axis',(0.,0.,1.));
#35082=DIRECTION('ref_axis',(1.,0.,0.));
#35083=DIRECTION('',(-1.,0.,0.));
#35084=DIRECTION('',(1.,0.,0.));
#35085=DIRECTION('center_axis',(0.,0.,-1.));
#35086=DIRECTION('ref_axis',(1.,0.,0.));
#35087=DIRECTION('center_axis',(0.,0.,-1.));
#35088=DIRECTION('ref_axis',(1.,0.,0.));
#35089=DIRECTION('center_axis',(0.,0.,-1.));
#35090=DIRECTION('ref_axis',(1.,0.,0.));
#35091=DIRECTION('center_axis',(0.,0.,-1.));
#35092=DIRECTION('ref_axis',(1.,0.,0.));
#35093=DIRECTION('center_axis',(0.,0.,-1.));
#35094=DIRECTION('ref_axis',(1.,0.,0.));
#35095=DIRECTION('center_axis',(0.,0.,-1.));
#35096=DIRECTION('ref_axis',(1.,0.,0.));
#35097=DIRECTION('center_axis',(0.,0.,-1.));
#35098=DIRECTION('ref_axis',(1.,0.,0.));
#35099=DIRECTION('center_axis',(0.,0.,-1.));
#35100=DIRECTION('ref_axis',(1.,0.,0.));
#35101=DIRECTION('center_axis',(0.,0.,-1.));
#35102=DIRECTION('ref_axis',(1.,0.,0.));
#35103=DIRECTION('center_axis',(0.,0.,-1.));
#35104=DIRECTION('ref_axis',(1.,0.,0.));
#35105=DIRECTION('center_axis',(0.,0.,-1.));
#35106=DIRECTION('ref_axis',(1.,0.,0.));
#35107=DIRECTION('center_axis',(0.,0.,-1.));
#35108=DIRECTION('ref_axis',(1.,0.,0.));
#35109=DIRECTION('center_axis',(0.,0.,-1.));
#35110=DIRECTION('ref_axis',(1.,0.,0.));
#35111=DIRECTION('center_axis',(0.,0.,-1.));
#35112=DIRECTION('ref_axis',(1.,0.,0.));
#35113=DIRECTION('center_axis',(0.,0.,-1.));
#35114=DIRECTION('ref_axis',(1.,0.,0.));
#35115=DIRECTION('center_axis',(0.,0.,-1.));
#35116=DIRECTION('ref_axis',(1.,0.,0.));
#35117=DIRECTION('center_axis',(0.,0.,-1.));
#35118=DIRECTION('ref_axis',(1.,0.,0.));
#35119=DIRECTION('center_axis',(0.,0.,-1.));
#35120=DIRECTION('ref_axis',(1.,0.,0.));
#35121=DIRECTION('center_axis',(0.,0.,-1.));
#35122=DIRECTION('ref_axis',(1.,0.,0.));
#35123=DIRECTION('center_axis',(0.,0.,-1.));
#35124=DIRECTION('ref_axis',(1.,0.,0.));
#35125=DIRECTION('center_axis',(0.,0.,-1.));
#35126=DIRECTION('ref_axis',(1.,0.,0.));
#35127=DIRECTION('center_axis',(0.,0.,1.));
#35128=DIRECTION('ref_axis',(1.,0.,0.));
#35129=DIRECTION('center_axis',(0.,0.,-1.));
#35130=DIRECTION('ref_axis',(1.,0.,0.));
#35131=DIRECTION('center_axis',(0.,0.,-1.));
#35132=DIRECTION('ref_axis',(1.,0.,0.));
#35133=DIRECTION('center_axis',(0.,0.,-1.));
#35134=DIRECTION('ref_axis',(1.,0.,0.));
#35135=DIRECTION('center_axis',(0.,0.,-1.));
#35136=DIRECTION('ref_axis',(1.,0.,0.));
#35137=DIRECTION('center_axis',(0.,0.,-1.));
#35138=DIRECTION('ref_axis',(1.,0.,0.));
#35139=DIRECTION('center_axis',(0.,0.,-1.));
#35140=DIRECTION('ref_axis',(1.,0.,0.));
#35141=DIRECTION('center_axis',(0.,0.,-1.));
#35142=DIRECTION('ref_axis',(1.,0.,0.));
#35143=DIRECTION('center_axis',(0.,0.,-1.));
#35144=DIRECTION('ref_axis',(1.,0.,0.));
#35145=DIRECTION('center_axis',(0.,0.,-1.));
#35146=DIRECTION('ref_axis',(1.,0.,0.));
#35147=DIRECTION('center_axis',(0.,0.,-1.));
#35148=DIRECTION('ref_axis',(1.,0.,0.));
#35149=DIRECTION('center_axis',(0.,0.,-1.));
#35150=DIRECTION('ref_axis',(1.,0.,0.));
#35151=DIRECTION('center_axis',(0.,0.,-1.));
#35152=DIRECTION('ref_axis',(1.,0.,0.));
#35153=DIRECTION('center_axis',(0.,0.,-1.));
#35154=DIRECTION('ref_axis',(1.,0.,0.));
#35155=DIRECTION('center_axis',(0.,0.,-1.));
#35156=DIRECTION('ref_axis',(1.,0.,0.));
#35157=DIRECTION('center_axis',(0.,0.,-1.));
#35158=DIRECTION('ref_axis',(1.,0.,0.));
#35159=DIRECTION('center_axis',(0.,0.,-1.));
#35160=DIRECTION('ref_axis',(1.,0.,0.));
#35161=DIRECTION('center_axis',(0.,0.,-1.));
#35162=DIRECTION('ref_axis',(1.,0.,0.));
#35163=DIRECTION('center_axis',(0.,0.,-1.));
#35164=DIRECTION('ref_axis',(1.,0.,0.));
#35165=DIRECTION('center_axis',(0.,0.,-1.));
#35166=DIRECTION('ref_axis',(1.,0.,0.));
#35167=DIRECTION('center_axis',(0.,0.,-1.));
#35168=DIRECTION('ref_axis',(1.,0.,0.));
#35169=DIRECTION('',(0.707106781186547,-8.65956056235493E-17,0.707106781186547));
#35170=DIRECTION('center_axis',(0.,0.,-1.));
#35171=DIRECTION('ref_axis',(1.,0.,0.));
#35172=DIRECTION('',(0.707106781186549,-8.65956056235495E-17,0.707106781186546));
#35173=DIRECTION('center_axis',(0.,0.,-1.));
#35174=DIRECTION('ref_axis',(1.,0.,0.));
#35175=DIRECTION('',(0.707106781186549,-8.65956056235495E-17,0.707106781186546));
#35176=DIRECTION('center_axis',(0.,0.,-1.));
#35177=DIRECTION('ref_axis',(1.,0.,0.));
#35178=DIRECTION('',(0.707106781186549,-8.65956056235495E-17,0.707106781186546));
#35179=DIRECTION('center_axis',(0.,0.,-1.));
#35180=DIRECTION('ref_axis',(1.,0.,0.));
#35181=DIRECTION('',(0.707106781186547,-8.65956056235493E-17,0.707106781186547));
#35182=DIRECTION('center_axis',(0.,0.,-1.));
#35183=DIRECTION('ref_axis',(1.,0.,0.));
#35184=DIRECTION('',(0.707106781186547,-8.65956056235493E-17,0.707106781186547));
#35185=DIRECTION('center_axis',(0.,0.,-1.));
#35186=DIRECTION('ref_axis',(1.,0.,0.));
#35187=DIRECTION('',(0.707106781186547,-8.65956056235493E-17,0.707106781186547));
#35188=DIRECTION('center_axis',(0.,0.,-1.));
#35189=DIRECTION('ref_axis',(1.,0.,0.));
#35190=DIRECTION('',(0.707106781186548,-8.65956056235493E-17,0.707106781186548));
#35191=DIRECTION('center_axis',(0.,0.,1.));
#35192=DIRECTION('ref_axis',(1.,0.,0.));
#35193=DIRECTION('center_axis',(0.,0.,-1.));
#35194=DIRECTION('ref_axis',(1.,0.,0.));
#35195=DIRECTION('center_axis',(0.,0.,-1.));
#35196=DIRECTION('ref_axis',(1.,0.,0.));
#35197=DIRECTION('',(0.,0.,-1.));
#35198=DIRECTION('center_axis',(0.,0.,-1.));
#35199=DIRECTION('ref_axis',(1.,0.,0.));
#35200=DIRECTION('',(0.707106781186548,-8.65956056235493E-17,0.707106781186548));
#35201=DIRECTION('center_axis',(0.,0.,1.));
#35202=DIRECTION('ref_axis',(1.,0.,0.));
#35203=DIRECTION('center_axis',(0.,0.,-1.));
#35204=DIRECTION('ref_axis',(1.,0.,0.));
#35205=DIRECTION('center_axis',(0.,0.,-1.));
#35206=DIRECTION('ref_axis',(1.,0.,0.));
#35207=DIRECTION('',(0.,0.,-1.));
#35208=DIRECTION('center_axis',(0.,0.,-1.));
#35209=DIRECTION('ref_axis',(1.,0.,0.));
#35210=DIRECTION('',(0.707106781186547,-8.65956056235493E-17,0.707106781186547));
#35211=DIRECTION('center_axis',(0.,0.,-1.));
#35212=DIRECTION('ref_axis',(1.,0.,0.));
#35213=DIRECTION('',(0.707106781186547,-8.65956056235493E-17,0.707106781186547));
#35214=DIRECTION('center_axis',(0.,0.707106781186541,-0.707106781186554));
#35215=DIRECTION('ref_axis',(-1.,0.,0.));
#35216=DIRECTION('',(1.,0.,0.));
#35217=DIRECTION('center_axis',(0.,-0.707106781186541,-0.707106781186554));
#35218=DIRECTION('ref_axis',(-1.,0.,0.));
#35219=DIRECTION('',(-1.,0.,0.));
#35220=DIRECTION('center_axis',(0.,1.,0.));
#35221=DIRECTION('ref_axis',(-1.,0.,0.));
#35222=DIRECTION('',(-1.,0.,0.));
#35223=DIRECTION('center_axis',(0.,0.,-1.));
#35224=DIRECTION('ref_axis',(1.,0.,0.));
#35225=DIRECTION('',(0.707106781186548,-8.65956056235493E-17,0.707106781186548));
#35226=DIRECTION('center_axis',(0.,0.,1.));
#35227=DIRECTION('ref_axis',(1.,0.,0.));
#35228=DIRECTION('center_axis',(0.,0.,-1.));
#35229=DIRECTION('ref_axis',(1.,0.,0.));
#35230=DIRECTION('center_axis',(0.,0.,-1.));
#35231=DIRECTION('ref_axis',(1.,0.,0.));
#35232=DIRECTION('',(0.,0.,-1.));
#35233=DIRECTION('center_axis',(0.,0.,-1.));
#35234=DIRECTION('ref_axis',(1.,0.,0.));
#35235=DIRECTION('',(0.707106781186548,-8.65956056235493E-17,0.707106781186548));
#35236=DIRECTION('center_axis',(0.,0.,1.));
#35237=DIRECTION('ref_axis',(1.,0.,0.));
#35238=DIRECTION('center_axis',(0.,0.,-1.));
#35239=DIRECTION('ref_axis',(1.,0.,0.));
#35240=DIRECTION('center_axis',(0.,0.,-1.));
#35241=DIRECTION('ref_axis',(1.,0.,0.));
#35242=DIRECTION('',(0.,0.,-1.));
#35243=DIRECTION('center_axis',(0.,0.,-1.));
#35244=DIRECTION('ref_axis',(1.,0.,0.));
#35245=DIRECTION('',(0.707106781186547,-8.65956056235493E-17,0.707106781186547));
#35246=DIRECTION('center_axis',(0.,0.,1.));
#35247=DIRECTION('ref_axis',(1.,0.,0.));
#35248=DIRECTION('center_axis',(0.,0.,-1.));
#35249=DIRECTION('ref_axis',(1.,0.,0.));
#35250=DIRECTION('center_axis',(0.,0.,-1.));
#35251=DIRECTION('ref_axis',(1.,0.,0.));
#35252=DIRECTION('',(0.,0.,-1.));
#35253=DIRECTION('center_axis',(0.,0.,-1.));
#35254=DIRECTION('ref_axis',(1.,0.,0.));
#35255=DIRECTION('',(0.707106781186548,-8.65956056235493E-17,0.707106781186548));
#35256=DIRECTION('center_axis',(0.,0.,1.));
#35257=DIRECTION('ref_axis',(1.,0.,0.));
#35258=DIRECTION('center_axis',(0.,0.,-1.));
#35259=DIRECTION('ref_axis',(1.,0.,0.));
#35260=DIRECTION('center_axis',(0.,0.,-1.));
#35261=DIRECTION('ref_axis',(1.,0.,0.));
#35262=DIRECTION('',(0.,0.,-1.));
#35263=DIRECTION('center_axis',(0.,0.,-1.));
#35264=DIRECTION('ref_axis',(1.,0.,0.));
#35265=DIRECTION('',(0.707106781186549,-8.65956056235495E-17,0.707106781186546));
#35266=DIRECTION('center_axis',(0.,0.,1.));
#35267=DIRECTION('ref_axis',(1.,0.,0.));
#35268=DIRECTION('center_axis',(0.,0.,-1.));
#35269=DIRECTION('ref_axis',(1.,0.,0.));
#35270=DIRECTION('center_axis',(0.,0.,-1.));
#35271=DIRECTION('ref_axis',(1.,0.,0.));
#35272=DIRECTION('',(0.,0.,-1.));
#35273=DIRECTION('center_axis',(0.,0.,-1.));
#35274=DIRECTION('ref_axis',(1.,0.,0.));
#35275=DIRECTION('',(0.707106781186549,-8.65956056235495E-17,0.707106781186546));
#35276=DIRECTION('center_axis',(0.,0.,1.));
#35277=DIRECTION('ref_axis',(1.,0.,0.));
#35278=DIRECTION('center_axis',(0.,0.,-1.));
#35279=DIRECTION('ref_axis',(1.,0.,0.));
#35280=DIRECTION('center_axis',(0.,0.,-1.));
#35281=DIRECTION('ref_axis',(1.,0.,0.));
#35282=DIRECTION('',(0.,0.,-1.));
#35283=DIRECTION('center_axis',(0.,0.,-1.));
#35284=DIRECTION('ref_axis',(1.,0.,0.));
#35285=DIRECTION('',(0.707106781186549,-8.65956056235495E-17,0.707106781186546));
#35286=DIRECTION('center_axis',(0.,0.,1.));
#35287=DIRECTION('ref_axis',(1.,0.,0.));
#35288=DIRECTION('center_axis',(0.,0.,-1.));
#35289=DIRECTION('ref_axis',(1.,0.,0.));
#35290=DIRECTION('center_axis',(0.,0.,-1.));
#35291=DIRECTION('ref_axis',(1.,0.,0.));
#35292=DIRECTION('',(0.,0.,-1.));
#35293=DIRECTION('center_axis',(0.,0.,-1.));
#35294=DIRECTION('ref_axis',(1.,0.,0.));
#35295=DIRECTION('',(0.707106781186549,-8.65956056235495E-17,0.707106781186546));
#35296=DIRECTION('center_axis',(0.,0.,1.));
#35297=DIRECTION('ref_axis',(1.,0.,0.));
#35298=DIRECTION('center_axis',(0.,0.,-1.));
#35299=DIRECTION('ref_axis',(1.,0.,0.));
#35300=DIRECTION('center_axis',(0.,0.,-1.));
#35301=DIRECTION('ref_axis',(1.,0.,0.));
#35302=DIRECTION('',(0.,0.,-1.));
#35303=DIRECTION('center_axis',(0.,0.,-1.));
#35304=DIRECTION('ref_axis',(1.,0.,0.));
#35305=DIRECTION('',(0.707106781186548,-8.65956056235493E-17,0.707106781186548));
#35306=DIRECTION('center_axis',(0.,0.,1.));
#35307=DIRECTION('ref_axis',(1.,0.,0.));
#35308=DIRECTION('center_axis',(0.,0.,-1.));
#35309=DIRECTION('ref_axis',(1.,0.,0.));
#35310=DIRECTION('center_axis',(0.,0.,-1.));
#35311=DIRECTION('ref_axis',(1.,0.,0.));
#35312=DIRECTION('',(0.,0.,-1.));
#35313=DIRECTION('center_axis',(0.,0.,-1.));
#35314=DIRECTION('ref_axis',(1.,0.,0.));
#35315=DIRECTION('',(0.707106781186548,-8.65956056235493E-17,0.707106781186548));
#35316=DIRECTION('center_axis',(0.,0.,1.));
#35317=DIRECTION('ref_axis',(1.,0.,0.));
#35318=DIRECTION('center_axis',(0.,0.,-1.));
#35319=DIRECTION('ref_axis',(1.,0.,0.));
#35320=DIRECTION('center_axis',(0.,0.,-1.));
#35321=DIRECTION('ref_axis',(1.,0.,0.));
#35322=DIRECTION('',(0.,0.,-1.));
#35323=DIRECTION('center_axis',(0.,0.,-1.));
#35324=DIRECTION('ref_axis',(1.,0.,0.));
#35325=DIRECTION('',(0.707106781186547,-8.65956056235493E-17,0.707106781186547));
#35326=DIRECTION('center_axis',(0.,0.,1.));
#35327=DIRECTION('ref_axis',(1.,0.,0.));
#35328=DIRECTION('center_axis',(0.,0.,-1.));
#35329=DIRECTION('ref_axis',(1.,0.,0.));
#35330=DIRECTION('center_axis',(0.,0.,-1.));
#35331=DIRECTION('ref_axis',(1.,0.,0.));
#35332=DIRECTION('',(0.,0.,-1.));
#35333=DIRECTION('center_axis',(0.,0.,-1.));
#35334=DIRECTION('ref_axis',(1.,0.,0.));
#35335=DIRECTION('',(0.707106781186547,-8.65956056235493E-17,0.707106781186547));
#35336=DIRECTION('center_axis',(0.,0.,1.));
#35337=DIRECTION('ref_axis',(1.,0.,0.));
#35338=DIRECTION('center_axis',(0.,0.,-1.));
#35339=DIRECTION('ref_axis',(1.,0.,0.));
#35340=DIRECTION('center_axis',(0.,0.,-1.));
#35341=DIRECTION('ref_axis',(1.,0.,0.));
#35342=DIRECTION('',(0.,0.,-1.));
#35343=DIRECTION('center_axis',(0.,0.,-1.));
#35344=DIRECTION('ref_axis',(1.,0.,0.));
#35345=DIRECTION('',(0.707106781186548,-8.65956056235493E-17,0.707106781186548));
#35346=DIRECTION('center_axis',(0.,0.,-1.));
#35347=DIRECTION('ref_axis',(1.,0.,0.));
#35348=DIRECTION('',(0.707106781186549,-8.65956056235495E-17,0.707106781186546));
#35349=DIRECTION('center_axis',(0.,0.,-1.));
#35350=DIRECTION('ref_axis',(1.,0.,0.));
#35351=DIRECTION('',(0.707106781186549,-8.65956056235495E-17,0.707106781186546));
#35352=DIRECTION('center_axis',(0.,0.,1.));
#35353=DIRECTION('ref_axis',(1.,0.,0.));
#35354=DIRECTION('center_axis',(0.,0.,-1.));
#35355=DIRECTION('ref_axis',(1.,0.,0.));
#35356=DIRECTION('center_axis',(0.,0.,-1.));
#35357=DIRECTION('ref_axis',(1.,0.,0.));
#35358=DIRECTION('',(0.,0.,-1.));
#35359=DIRECTION('center_axis',(0.,0.,-1.));
#35360=DIRECTION('ref_axis',(1.,0.,0.));
#35361=DIRECTION('',(0.707106781186549,-8.65956056235495E-17,0.707106781186546));
#35362=DIRECTION('center_axis',(0.,0.,1.));
#35363=DIRECTION('ref_axis',(1.,0.,0.));
#35364=DIRECTION('center_axis',(0.,0.,-1.));
#35365=DIRECTION('ref_axis',(1.,0.,0.));
#35366=DIRECTION('center_axis',(0.,0.,-1.));
#35367=DIRECTION('ref_axis',(1.,0.,0.));
#35368=DIRECTION('',(0.,0.,-1.));
#35369=DIRECTION('center_axis',(0.,0.,-1.));
#35370=DIRECTION('ref_axis',(1.,0.,0.));
#35371=DIRECTION('',(0.707106781186547,-8.65956056235493E-17,0.707106781186547));
#35372=DIRECTION('center_axis',(0.,0.,1.));
#35373=DIRECTION('ref_axis',(1.,0.,0.));
#35374=DIRECTION('center_axis',(0.,0.,-1.));
#35375=DIRECTION('ref_axis',(1.,0.,0.));
#35376=DIRECTION('center_axis',(0.,0.,-1.));
#35377=DIRECTION('ref_axis',(1.,0.,0.));
#35378=DIRECTION('',(0.,0.,-1.));
#35379=DIRECTION('center_axis',(0.,0.,-1.));
#35380=DIRECTION('ref_axis',(1.,0.,0.));
#35381=DIRECTION('',(0.707106781186549,-8.65956056235495E-17,0.707106781186546));
#35382=DIRECTION('center_axis',(0.,0.,1.));
#35383=DIRECTION('ref_axis',(1.,0.,0.));
#35384=DIRECTION('center_axis',(0.,0.,-1.));
#35385=DIRECTION('ref_axis',(1.,0.,0.));
#35386=DIRECTION('center_axis',(0.,0.,-1.));
#35387=DIRECTION('ref_axis',(1.,0.,0.));
#35388=DIRECTION('',(0.,0.,-1.));
#35389=DIRECTION('center_axis',(0.,0.,-1.));
#35390=DIRECTION('ref_axis',(1.,0.,0.));
#35391=DIRECTION('',(0.707106781186548,-8.65956056235493E-17,0.707106781186548));
#35392=DIRECTION('center_axis',(0.,0.,1.));
#35393=DIRECTION('ref_axis',(1.,0.,0.));
#35394=DIRECTION('center_axis',(0.,0.,-1.));
#35395=DIRECTION('ref_axis',(1.,0.,0.));
#35396=DIRECTION('center_axis',(0.,0.,-1.));
#35397=DIRECTION('ref_axis',(1.,0.,0.));
#35398=DIRECTION('',(0.,0.,-1.));
#35399=DIRECTION('center_axis',(0.,0.,-1.));
#35400=DIRECTION('ref_axis',(1.,0.,0.));
#35401=DIRECTION('',(0.707106781186547,-8.65956056235493E-17,0.707106781186547));
#35402=DIRECTION('center_axis',(0.,0.,1.));
#35403=DIRECTION('ref_axis',(1.,0.,0.));
#35404=DIRECTION('center_axis',(0.,0.,-1.));
#35405=DIRECTION('ref_axis',(1.,0.,0.));
#35406=DIRECTION('center_axis',(0.,0.,-1.));
#35407=DIRECTION('ref_axis',(1.,0.,0.));
#35408=DIRECTION('',(0.,0.,-1.));
#35409=DIRECTION('center_axis',(0.,0.,-1.));
#35410=DIRECTION('ref_axis',(1.,0.,0.));
#35411=DIRECTION('',(0.707106781186547,-8.65956056235493E-17,0.707106781186547));
#35412=DIRECTION('center_axis',(0.,0.,1.));
#35413=DIRECTION('ref_axis',(1.,0.,0.));
#35414=DIRECTION('center_axis',(0.,0.,-1.));
#35415=DIRECTION('ref_axis',(1.,0.,0.));
#35416=DIRECTION('center_axis',(0.,0.,-1.));
#35417=DIRECTION('ref_axis',(1.,0.,0.));
#35418=DIRECTION('',(0.,0.,-1.));
#35419=DIRECTION('center_axis',(0.,0.,-1.));
#35420=DIRECTION('ref_axis',(1.,0.,0.));
#35421=DIRECTION('',(0.707106781186547,-8.65956056235493E-17,0.707106781186547));
#35422=DIRECTION('center_axis',(0.,0.,1.));
#35423=DIRECTION('ref_axis',(1.,0.,0.));
#35424=DIRECTION('center_axis',(0.,0.,-1.));
#35425=DIRECTION('ref_axis',(1.,0.,0.));
#35426=DIRECTION('center_axis',(0.,0.,-1.));
#35427=DIRECTION('ref_axis',(1.,0.,0.));
#35428=DIRECTION('',(0.,0.,-1.));
#35429=DIRECTION('center_axis',(0.,0.,-1.));
#35430=DIRECTION('ref_axis',(1.,0.,0.));
#35431=DIRECTION('',(0.707106781186547,-8.65956056235493E-17,0.707106781186547));
#35432=DIRECTION('center_axis',(0.,0.,1.));
#35433=DIRECTION('ref_axis',(1.,0.,0.));
#35434=DIRECTION('center_axis',(0.,0.,-1.));
#35435=DIRECTION('ref_axis',(1.,0.,0.));
#35436=DIRECTION('center_axis',(0.,0.,-1.));
#35437=DIRECTION('ref_axis',(1.,0.,0.));
#35438=DIRECTION('',(0.,0.,-1.));
#35439=DIRECTION('center_axis',(0.,0.,-1.));
#35440=DIRECTION('ref_axis',(1.,0.,0.));
#35441=DIRECTION('',(0.707106781186547,-8.65956056235493E-17,0.707106781186547));
#35442=DIRECTION('center_axis',(0.,0.,1.));
#35443=DIRECTION('ref_axis',(1.,0.,0.));
#35444=DIRECTION('center_axis',(0.,0.,-1.));
#35445=DIRECTION('ref_axis',(1.,0.,0.));
#35446=DIRECTION('center_axis',(0.,0.,-1.));
#35447=DIRECTION('ref_axis',(1.,0.,0.));
#35448=DIRECTION('',(0.,0.,-1.));
#35449=DIRECTION('center_axis',(0.,0.,-1.));
#35450=DIRECTION('ref_axis',(1.,0.,0.));
#35451=DIRECTION('',(0.707106781186549,-8.65956056235495E-17,0.707106781186546));
#35452=DIRECTION('center_axis',(0.,0.,1.));
#35453=DIRECTION('ref_axis',(1.,0.,0.));
#35454=DIRECTION('center_axis',(0.,0.,-1.));
#35455=DIRECTION('ref_axis',(1.,0.,0.));
#35456=DIRECTION('center_axis',(0.,0.,-1.));
#35457=DIRECTION('ref_axis',(1.,0.,0.));
#35458=DIRECTION('',(0.,0.,-1.));
#35459=DIRECTION('center_axis',(0.,0.,-1.));
#35460=DIRECTION('ref_axis',(1.,0.,0.));
#35461=DIRECTION('',(0.707106781186547,-8.65956056235493E-17,0.707106781186547));
#35462=DIRECTION('center_axis',(0.,0.,1.));
#35463=DIRECTION('ref_axis',(1.,0.,0.));
#35464=DIRECTION('center_axis',(0.,0.,-1.));
#35465=DIRECTION('ref_axis',(1.,0.,0.));
#35466=DIRECTION('center_axis',(0.,0.,-1.));
#35467=DIRECTION('ref_axis',(1.,0.,0.));
#35468=DIRECTION('',(0.,0.,-1.));
#35469=DIRECTION('center_axis',(0.,0.,-1.));
#35470=DIRECTION('ref_axis',(1.,0.,0.));
#35471=DIRECTION('',(0.707106781186549,-8.65956056235495E-17,0.707106781186546));
#35472=DIRECTION('center_axis',(0.,0.,1.));
#35473=DIRECTION('ref_axis',(1.,0.,0.));
#35474=DIRECTION('center_axis',(0.,0.,-1.));
#35475=DIRECTION('ref_axis',(1.,0.,0.));
#35476=DIRECTION('center_axis',(0.,0.,-1.));
#35477=DIRECTION('ref_axis',(1.,0.,0.));
#35478=DIRECTION('',(0.,0.,-1.));
#35479=DIRECTION('center_axis',(0.,0.,-1.));
#35480=DIRECTION('ref_axis',(1.,0.,0.));
#35481=DIRECTION('',(0.707106781186549,-8.65956056235495E-17,0.707106781186546));
#35482=DIRECTION('center_axis',(0.,0.,1.));
#35483=DIRECTION('ref_axis',(1.,0.,0.));
#35484=DIRECTION('center_axis',(0.,0.,-1.));
#35485=DIRECTION('ref_axis',(1.,0.,0.));
#35486=DIRECTION('center_axis',(0.,0.,-1.));
#35487=DIRECTION('ref_axis',(1.,0.,0.));
#35488=DIRECTION('',(0.,0.,-1.));
#35489=DIRECTION('center_axis',(0.,0.,-1.));
#35490=DIRECTION('ref_axis',(1.,0.,0.));
#35491=DIRECTION('',(0.707106781186547,-8.65956056235493E-17,0.707106781186547));
#35492=DIRECTION('center_axis',(0.,0.,1.));
#35493=DIRECTION('ref_axis',(1.,0.,0.));
#35494=DIRECTION('center_axis',(0.,0.,-1.));
#35495=DIRECTION('ref_axis',(1.,0.,0.));
#35496=DIRECTION('center_axis',(0.,0.,-1.));
#35497=DIRECTION('ref_axis',(1.,0.,0.));
#35498=DIRECTION('',(0.,0.,-1.));
#35499=DIRECTION('center_axis',(0.,-0.707106781186541,0.707106781186554));
#35500=DIRECTION('ref_axis',(1.,0.,0.));
#35501=DIRECTION('',(-1.,0.,0.));
#35502=DIRECTION('',(1.,0.,0.));
#35503=DIRECTION('center_axis',(0.,0.707106781186541,0.707106781186554));
#35504=DIRECTION('ref_axis',(1.,0.,0.));
#35505=DIRECTION('',(1.,0.,0.));
#35506=DIRECTION('center_axis',(0.,0.,1.));
#35507=DIRECTION('ref_axis',(1.,0.,0.));
#35508=DIRECTION('center_axis',(0.,0.,1.));
#35509=DIRECTION('ref_axis',(1.,0.,0.));
#35510=DIRECTION('center_axis',(0.,0.,1.));
#35511=DIRECTION('ref_axis',(1.,0.,0.));
#35512=DIRECTION('center_axis',(0.,0.,1.));
#35513=DIRECTION('ref_axis',(1.,0.,0.));
#35514=DIRECTION('center_axis',(0.,0.,1.));
#35515=DIRECTION('ref_axis',(1.,0.,0.));
#35516=DIRECTION('center_axis',(0.,0.,1.));
#35517=DIRECTION('ref_axis',(1.,0.,0.));
#35518=DIRECTION('center_axis',(0.,0.,1.));
#35519=DIRECTION('ref_axis',(1.,0.,0.));
#35520=DIRECTION('center_axis',(0.,0.,1.));
#35521=DIRECTION('ref_axis',(1.,0.,0.));
#35522=DIRECTION('center_axis',(0.,0.,1.));
#35523=DIRECTION('ref_axis',(1.,0.,0.));
#35524=DIRECTION('center_axis',(0.,0.,1.));
#35525=DIRECTION('ref_axis',(1.,0.,0.));
#35526=DIRECTION('center_axis',(0.,0.,1.));
#35527=DIRECTION('ref_axis',(1.,0.,0.));
#35528=DIRECTION('center_axis',(0.,0.,1.));
#35529=DIRECTION('ref_axis',(1.,0.,0.));
#35530=DIRECTION('center_axis',(0.,0.,1.));
#35531=DIRECTION('ref_axis',(1.,0.,0.));
#35532=DIRECTION('center_axis',(0.,0.,1.));
#35533=DIRECTION('ref_axis',(1.,0.,0.));
#35534=DIRECTION('center_axis',(0.,0.,1.));
#35535=DIRECTION('ref_axis',(1.,0.,0.));
#35536=DIRECTION('center_axis',(0.,0.,1.));
#35537=DIRECTION('ref_axis',(1.,0.,0.));
#35538=DIRECTION('center_axis',(0.,0.,1.));
#35539=DIRECTION('ref_axis',(1.,0.,0.));
#35540=DIRECTION('center_axis',(0.,0.,1.));
#35541=DIRECTION('ref_axis',(1.,0.,0.));
#35542=DIRECTION('center_axis',(0.,0.,1.));
#35543=DIRECTION('ref_axis',(1.,0.,0.));
#35544=DIRECTION('center_axis',(0.,0.,1.));
#35545=DIRECTION('ref_axis',(1.,0.,0.));
#35546=DIRECTION('center_axis',(0.,0.,1.));
#35547=DIRECTION('ref_axis',(1.,0.,0.));
#35548=DIRECTION('center_axis',(0.,0.,1.));
#35549=DIRECTION('ref_axis',(1.,0.,0.));
#35550=DIRECTION('center_axis',(0.,0.,1.));
#35551=DIRECTION('ref_axis',(1.,0.,0.));
#35552=DIRECTION('center_axis',(0.,0.,1.));
#35553=DIRECTION('ref_axis',(1.,0.,0.));
#35554=DIRECTION('center_axis',(0.,0.,1.));
#35555=DIRECTION('ref_axis',(1.,0.,0.));
#35556=DIRECTION('center_axis',(0.,0.,1.));
#35557=DIRECTION('ref_axis',(1.,0.,0.));
#35558=DIRECTION('center_axis',(0.,0.,1.));
#35559=DIRECTION('ref_axis',(1.,0.,0.));
#35560=DIRECTION('center_axis',(0.,0.,1.));
#35561=DIRECTION('ref_axis',(1.,0.,0.));
#35562=DIRECTION('center_axis',(0.,0.,1.));
#35563=DIRECTION('ref_axis',(1.,0.,0.));
#35564=DIRECTION('center_axis',(0.,0.,1.));
#35565=DIRECTION('ref_axis',(1.,0.,0.));
#35566=DIRECTION('center_axis',(0.,0.,1.));
#35567=DIRECTION('ref_axis',(1.,0.,0.));
#35568=DIRECTION('center_axis',(0.,0.,1.));
#35569=DIRECTION('ref_axis',(1.,0.,0.));
#35570=DIRECTION('center_axis',(0.,0.,1.));
#35571=DIRECTION('ref_axis',(1.,0.,0.));
#35572=DIRECTION('center_axis',(0.,0.,1.));
#35573=DIRECTION('ref_axis',(1.,0.,0.));
#35574=DIRECTION('center_axis',(0.,0.,1.));
#35575=DIRECTION('ref_axis',(1.,0.,0.));
#35576=DIRECTION('center_axis',(0.,0.,1.));
#35577=DIRECTION('ref_axis',(1.,0.,0.));
#35578=DIRECTION('center_axis',(0.,0.,1.));
#35579=DIRECTION('ref_axis',(1.,0.,0.));
#35580=DIRECTION('center_axis',(0.,0.,1.));
#35581=DIRECTION('ref_axis',(1.,0.,0.));
#35582=DIRECTION('center_axis',(0.,0.,1.));
#35583=DIRECTION('ref_axis',(1.,0.,0.));
#35584=DIRECTION('center_axis',(0.,0.,1.));
#35585=DIRECTION('ref_axis',(1.,0.,0.));
#35586=DIRECTION('center_axis',(0.,0.,1.));
#35587=DIRECTION('ref_axis',(1.,0.,0.));
#35588=DIRECTION('center_axis',(0.,0.,1.));
#35589=DIRECTION('ref_axis',(1.,0.,0.));
#35590=DIRECTION('center_axis',(0.,0.,1.));
#35591=DIRECTION('ref_axis',(1.,0.,0.));
#35592=DIRECTION('center_axis',(0.,0.,1.));
#35593=DIRECTION('ref_axis',(1.,0.,0.));
#35594=DIRECTION('',(0.707106781186547,8.65956056235493E-17,-0.707106781186547));
#35595=DIRECTION('center_axis',(0.,0.,1.));
#35596=DIRECTION('ref_axis',(1.,0.,0.));
#35597=DIRECTION('',(0.707106781186547,8.65956056235493E-17,-0.707106781186547));
#35598=DIRECTION('center_axis',(0.,0.,1.));
#35599=DIRECTION('ref_axis',(1.,0.,0.));
#35600=DIRECTION('',(0.707106781186549,8.65956056235495E-17,-0.707106781186546));
#35601=DIRECTION('center_axis',(0.,0.,1.));
#35602=DIRECTION('ref_axis',(1.,0.,0.));
#35603=DIRECTION('',(0.707106781186549,8.65956056235495E-17,-0.707106781186546));
#35604=DIRECTION('center_axis',(0.,0.,1.));
#35605=DIRECTION('ref_axis',(1.,0.,0.));
#35606=DIRECTION('',(0.707106781186547,8.65956056235493E-17,-0.707106781186547));
#35607=DIRECTION('center_axis',(0.,0.,1.));
#35608=DIRECTION('ref_axis',(1.,0.,0.));
#35609=DIRECTION('',(0.707106781186549,8.65956056235495E-17,-0.707106781186546));
#35610=DIRECTION('center_axis',(0.,0.,1.));
#35611=DIRECTION('ref_axis',(1.,0.,0.));
#35612=DIRECTION('',(0.707106781186547,8.65956056235493E-17,-0.707106781186547));
#35613=DIRECTION('center_axis',(0.,0.,1.));
#35614=DIRECTION('ref_axis',(1.,0.,0.));
#35615=DIRECTION('',(0.707106781186547,8.65956056235493E-17,-0.707106781186547));
#35616=DIRECTION('center_axis',(0.,0.,1.));
#35617=DIRECTION('ref_axis',(1.,0.,0.));
#35618=DIRECTION('',(0.707106781186548,8.65956056235494E-17,-0.707106781186548));
#35619=DIRECTION('center_axis',(0.,0.,-1.));
#35620=DIRECTION('ref_axis',(1.,0.,0.));
#35621=DIRECTION('center_axis',(0.,0.,-1.));
#35622=DIRECTION('ref_axis',(1.,0.,0.));
#35623=DIRECTION('',(0.,0.,-1.));
#35624=DIRECTION('center_axis',(0.,0.,1.));
#35625=DIRECTION('ref_axis',(1.,0.,0.));
#35626=DIRECTION('',(0.707106781186548,8.65956056235494E-17,-0.707106781186548));
#35627=DIRECTION('center_axis',(0.,0.,-1.));
#35628=DIRECTION('ref_axis',(1.,0.,0.));
#35629=DIRECTION('center_axis',(0.,0.,-1.));
#35630=DIRECTION('ref_axis',(1.,0.,0.));
#35631=DIRECTION('',(0.,0.,-1.));
#35632=DIRECTION('center_axis',(0.,0.,1.));
#35633=DIRECTION('ref_axis',(1.,0.,0.));
#35634=DIRECTION('',(0.707106781186547,8.65956056235493E-17,-0.707106781186547));
#35635=DIRECTION('center_axis',(0.,0.,-1.));
#35636=DIRECTION('ref_axis',(1.,0.,0.));
#35637=DIRECTION('center_axis',(0.,0.,-1.));
#35638=DIRECTION('ref_axis',(1.,0.,0.));
#35639=DIRECTION('',(0.,0.,-1.));
#35640=DIRECTION('center_axis',(0.,0.,1.));
#35641=DIRECTION('ref_axis',(1.,0.,0.));
#35642=DIRECTION('',(0.707106781186548,8.65956056235494E-17,-0.707106781186548));
#35643=DIRECTION('center_axis',(0.,0.,-1.));
#35644=DIRECTION('ref_axis',(1.,0.,0.));
#35645=DIRECTION('center_axis',(0.,0.,-1.));
#35646=DIRECTION('ref_axis',(1.,0.,0.));
#35647=DIRECTION('',(0.,0.,-1.));
#35648=DIRECTION('center_axis',(0.,0.,1.));
#35649=DIRECTION('ref_axis',(1.,0.,0.));
#35650=DIRECTION('',(0.707106781186549,8.65956056235495E-17,-0.707106781186546));
#35651=DIRECTION('center_axis',(0.,0.,-1.));
#35652=DIRECTION('ref_axis',(1.,0.,0.));
#35653=DIRECTION('center_axis',(0.,0.,-1.));
#35654=DIRECTION('ref_axis',(1.,0.,0.));
#35655=DIRECTION('',(0.,0.,-1.));
#35656=DIRECTION('center_axis',(0.,0.,1.));
#35657=DIRECTION('ref_axis',(1.,0.,0.));
#35658=DIRECTION('',(0.707106781186549,8.65956056235495E-17,-0.707106781186546));
#35659=DIRECTION('center_axis',(0.,0.,-1.));
#35660=DIRECTION('ref_axis',(1.,0.,0.));
#35661=DIRECTION('center_axis',(0.,0.,-1.));
#35662=DIRECTION('ref_axis',(1.,0.,0.));
#35663=DIRECTION('',(0.,0.,-1.));
#35664=DIRECTION('center_axis',(0.,0.,1.));
#35665=DIRECTION('ref_axis',(1.,0.,0.));
#35666=DIRECTION('',(0.707106781186549,8.65956056235495E-17,-0.707106781186546));
#35667=DIRECTION('center_axis',(0.,0.,-1.));
#35668=DIRECTION('ref_axis',(1.,0.,0.));
#35669=DIRECTION('center_axis',(0.,0.,-1.));
#35670=DIRECTION('ref_axis',(1.,0.,0.));
#35671=DIRECTION('',(0.,0.,-1.));
#35672=DIRECTION('center_axis',(0.,0.,1.));
#35673=DIRECTION('ref_axis',(1.,0.,0.));
#35674=DIRECTION('',(0.707106781186548,8.65956056235494E-17,-0.707106781186548));
#35675=DIRECTION('center_axis',(0.,0.,-1.));
#35676=DIRECTION('ref_axis',(1.,0.,0.));
#35677=DIRECTION('center_axis',(0.,0.,-1.));
#35678=DIRECTION('ref_axis',(1.,0.,0.));
#35679=DIRECTION('',(0.,0.,-1.));
#35680=DIRECTION('center_axis',(0.,0.,1.));
#35681=DIRECTION('ref_axis',(1.,0.,0.));
#35682=DIRECTION('',(0.707106781186547,8.65956056235493E-17,-0.707106781186547));
#35683=DIRECTION('center_axis',(0.,0.,-1.));
#35684=DIRECTION('ref_axis',(1.,0.,0.));
#35685=DIRECTION('center_axis',(0.,0.,-1.));
#35686=DIRECTION('ref_axis',(1.,0.,0.));
#35687=DIRECTION('',(0.,0.,-1.));
#35688=DIRECTION('center_axis',(0.,0.,1.));
#35689=DIRECTION('ref_axis',(1.,0.,0.));
#35690=DIRECTION('',(0.707106781186548,8.65956056235494E-17,-0.707106781186548));
#35691=DIRECTION('center_axis',(0.,0.,-1.));
#35692=DIRECTION('ref_axis',(1.,0.,0.));
#35693=DIRECTION('center_axis',(0.,0.,-1.));
#35694=DIRECTION('ref_axis',(1.,0.,0.));
#35695=DIRECTION('',(0.,0.,-1.));
#35696=DIRECTION('center_axis',(0.,0.,1.));
#35697=DIRECTION('ref_axis',(1.,0.,0.));
#35698=DIRECTION('',(0.707106781186547,8.65956056235493E-17,-0.707106781186547));
#35699=DIRECTION('center_axis',(0.,0.,1.));
#35700=DIRECTION('ref_axis',(1.,0.,0.));
#35701=DIRECTION('',(0.707106781186547,8.65956056235493E-17,-0.707106781186547));
#35702=DIRECTION('center_axis',(0.,0.,1.));
#35703=DIRECTION('ref_axis',(1.,0.,0.));
#35704=DIRECTION('',(0.707106781186547,8.65956056235493E-17,-0.707106781186547));
#35705=DIRECTION('center_axis',(0.,0.,1.));
#35706=DIRECTION('ref_axis',(1.,0.,0.));
#35707=DIRECTION('',(0.707106781186548,8.65956056235493E-17,-0.707106781186548));
#35708=DIRECTION('center_axis',(0.,0.,1.));
#35709=DIRECTION('ref_axis',(1.,0.,0.));
#35710=DIRECTION('',(0.707106781186549,8.65956056235495E-17,-0.707106781186546));
#35711=DIRECTION('center_axis',(0.,0.,1.));
#35712=DIRECTION('ref_axis',(1.,0.,0.));
#35713=DIRECTION('',(0.707106781186547,8.65956056235493E-17,-0.707106781186547));
#35714=DIRECTION('center_axis',(0.,0.,1.));
#35715=DIRECTION('ref_axis',(1.,0.,0.));
#35716=DIRECTION('',(0.707106781186549,8.65956056235495E-17,-0.707106781186546));
#35717=DIRECTION('center_axis',(0.,0.,1.));
#35718=DIRECTION('ref_axis',(1.,0.,0.));
#35719=DIRECTION('',(0.707106781186549,8.65956056235495E-17,-0.707106781186546));
#35720=DIRECTION('center_axis',(0.,0.,1.));
#35721=DIRECTION('ref_axis',(1.,0.,0.));
#35722=DIRECTION('',(0.707106781186548,8.65956056235493E-17,-0.707106781186548));
#35723=DIRECTION('center_axis',(0.,0.,1.));
#35724=DIRECTION('ref_axis',(1.,0.,0.));
#35725=DIRECTION('',(0.707106781186548,8.65956056235493E-17,-0.707106781186548));
#35726=DIRECTION('center_axis',(0.,0.,1.));
#35727=DIRECTION('ref_axis',(1.,0.,0.));
#35728=DIRECTION('',(0.707106781186547,8.65956056235493E-17,-0.707106781186547));
#35729=DIRECTION('center_axis',(0.,0.,1.));
#35730=DIRECTION('ref_axis',(1.,0.,0.));
#35731=DIRECTION('',(0.707106781186548,8.65956056235493E-17,-0.707106781186548));
#35732=DIRECTION('center_axis',(0.,0.,1.));
#35733=DIRECTION('ref_axis',(1.,0.,0.));
#35734=DIRECTION('',(0.707106781186549,8.65956056235495E-17,-0.707106781186546));
#35735=DIRECTION('center_axis',(0.,0.,1.));
#35736=DIRECTION('ref_axis',(1.,0.,0.));
#35737=DIRECTION('',(0.707106781186549,8.65956056235495E-17,-0.707106781186546));
#35738=DIRECTION('center_axis',(0.,0.,1.));
#35739=DIRECTION('ref_axis',(1.,0.,0.));
#35740=DIRECTION('',(0.707106781186549,8.65956056235495E-17,-0.707106781186546));
#35741=DIRECTION('center_axis',(0.,0.,1.));
#35742=DIRECTION('ref_axis',(1.,0.,0.));
#35743=DIRECTION('',(0.707106781186549,8.65956056235495E-17,-0.707106781186546));
#35744=DIRECTION('center_axis',(0.,0.,1.));
#35745=DIRECTION('ref_axis',(1.,0.,0.));
#35746=DIRECTION('',(0.707106781186548,8.65956056235493E-17,-0.707106781186548));
#35747=DIRECTION('center_axis',(0.,0.,1.));
#35748=DIRECTION('ref_axis',(1.,0.,0.));
#35749=DIRECTION('',(0.707106781186548,8.65956056235493E-17,-0.707106781186548));
#35750=DIRECTION('center_axis',(0.,0.,1.));
#35751=DIRECTION('ref_axis',(1.,0.,0.));
#35752=DIRECTION('',(0.707106781186547,8.65956056235493E-17,-0.707106781186547));
#35753=DIRECTION('center_axis',(0.,0.,1.));
#35754=DIRECTION('ref_axis',(1.,0.,0.));
#35755=DIRECTION('',(0.707106781186547,8.65956056235493E-17,-0.707106781186547));
#35756=DIRECTION('center_axis',(0.,0.,1.));
#35757=DIRECTION('ref_axis',(1.,0.,0.));
#35758=DIRECTION('',(0.707106781186548,8.65956056235493E-17,-0.707106781186548));
#35759=DIRECTION('center_axis',(0.,0.,1.));
#35760=DIRECTION('ref_axis',(1.,0.,0.));
#35761=DIRECTION('',(0.707106781186548,8.65956056235493E-17,-0.707106781186548));
#35762=DIRECTION('center_axis',(0.,0.,1.));
#35763=DIRECTION('ref_axis',(1.,0.,0.));
#35764=DIRECTION('',(0.707106781186547,8.65956056235493E-17,-0.707106781186547));
#35765=DIRECTION('center_axis',(0.,0.,-1.));
#35766=DIRECTION('ref_axis',(1.,0.,0.));
#35767=DIRECTION('center_axis',(0.,0.,-1.));
#35768=DIRECTION('ref_axis',(1.,0.,0.));
#35769=DIRECTION('',(0.,0.,-1.));
#35770=DIRECTION('center_axis',(0.,0.,1.));
#35771=DIRECTION('ref_axis',(1.,0.,0.));
#35772=DIRECTION('',(0.707106781186549,8.65956056235495E-17,-0.707106781186546));
#35773=DIRECTION('center_axis',(0.,0.,-1.));
#35774=DIRECTION('ref_axis',(1.,0.,0.));
#35775=DIRECTION('center_axis',(0.,0.,-1.));
#35776=DIRECTION('ref_axis',(1.,0.,0.));
#35777=DIRECTION('',(0.,0.,-1.));
#35778=DIRECTION('center_axis',(0.,0.,1.));
#35779=DIRECTION('ref_axis',(1.,0.,0.));
#35780=DIRECTION('',(0.,0.,1.));
#35781=DIRECTION('center_axis',(0.,-1.,0.));
#35782=DIRECTION('ref_axis',(1.,0.,0.));
#43740=CARTESIAN_POINT('',(0.,0.,0.));
#43741=CARTESIAN_POINT('Origin',(18.75,18.75,48.25));
#43742=CARTESIAN_POINT('',(14.25,18.75,48.));
#43743=CARTESIAN_POINT('Origin',(18.75,18.75,48.));
#43744=CARTESIAN_POINT('',(13.75,18.75,48.5));
#43745=CARTESIAN_POINT('',(14.,18.75,48.25));
#43746=CARTESIAN_POINT('Origin',(18.75,18.75,48.5));
#43747=CARTESIAN_POINT('Origin',(18.75,18.75,57.));
#43748=CARTESIAN_POINT('',(14.25,18.75,43.25));
#43749=CARTESIAN_POINT('',(14.25,18.75,57.));
#43750=CARTESIAN_POINT('Origin',(18.75,18.75,43.25));
#43751=CARTESIAN_POINT('Origin',(18.75,18.75,48.5));
#43752=CARTESIAN_POINT('',(11.75,18.75,48.5));
#43753=CARTESIAN_POINT('Origin',(18.75,18.75,48.5));
#43754=CARTESIAN_POINT('Origin',(-56.25,-18.75,48.25));
#43755=CARTESIAN_POINT('',(-60.75,-18.75,48.));
#43756=CARTESIAN_POINT('Origin',(-56.25,-18.75,48.));
#43757=CARTESIAN_POINT('',(-61.25,-18.75,48.5));
#43758=CARTESIAN_POINT('',(-61.,-18.75,48.25));
#43759=CARTESIAN_POINT('Origin',(-56.25,-18.75,48.5));
#43760=CARTESIAN_POINT('Origin',(-56.25,-18.75,57.));
#43761=CARTESIAN_POINT('',(-60.75,-18.75,43.25));
#43762=CARTESIAN_POINT('',(-60.75,-18.75,57.));
#43763=CARTESIAN_POINT('Origin',(-56.25,-18.75,43.25));
#43764=CARTESIAN_POINT('Origin',(-56.25,-18.75,48.5));
#43765=CARTESIAN_POINT('',(-63.25,-18.75,48.5));
#43766=CARTESIAN_POINT('Origin',(-56.25,-18.75,48.5));
#43767=CARTESIAN_POINT('Origin',(-18.75,18.75,48.25));
#43768=CARTESIAN_POINT('',(-23.25,18.75,48.));
#43769=CARTESIAN_POINT('Origin',(-18.75,18.75,48.));
#43770=CARTESIAN_POINT('',(-23.75,18.75,48.5));
#43771=CARTESIAN_POINT('',(-23.5,18.75,48.25));
#43772=CARTESIAN_POINT('Origin',(-18.75,18.75,48.5));
#43773=CARTESIAN_POINT('Origin',(-18.75,18.75,57.));
#43774=CARTESIAN_POINT('',(-23.25,18.75,43.25));
#43775=CARTESIAN_POINT('',(-23.25,18.75,57.));
#43776=CARTESIAN_POINT('Origin',(-18.75,18.75,43.25));
#43777=CARTESIAN_POINT('Origin',(-18.75,18.75,48.5));
#43778=CARTESIAN_POINT('',(-25.75,18.75,48.5));
#43779=CARTESIAN_POINT('Origin',(-18.75,18.75,48.5));
#43780=CARTESIAN_POINT('Origin',(-18.75,-56.25,48.25));
#43781=CARTESIAN_POINT('',(-23.25,-56.25,48.));
#43782=CARTESIAN_POINT('Origin',(-18.75,-56.25,48.));
#43783=CARTESIAN_POINT('',(-23.75,-56.25,48.5));
#43784=CARTESIAN_POINT('',(-23.5,-56.25,48.25));
#43785=CARTESIAN_POINT('Origin',(-18.75,-56.25,48.5));
#43786=CARTESIAN_POINT('Origin',(-18.75,-56.25,57.));
#43787=CARTESIAN_POINT('',(-23.25,-56.25,43.25));
#43788=CARTESIAN_POINT('',(-23.25,-56.25,57.));
#43789=CARTESIAN_POINT('Origin',(-18.75,-56.25,43.25));
#43790=CARTESIAN_POINT('Origin',(-18.75,-56.25,48.5));
#43791=CARTESIAN_POINT('',(-25.75,-56.25,48.5));
#43792=CARTESIAN_POINT('Origin',(-18.75,-56.25,48.5));
#43793=CARTESIAN_POINT('Origin',(-18.75,-18.75,48.25));
#43794=CARTESIAN_POINT('',(-23.25,-18.75,48.));
#43795=CARTESIAN_POINT('Origin',(-18.75,-18.75,48.));
#43796=CARTESIAN_POINT('',(-23.75,-18.75,48.5));
#43797=CARTESIAN_POINT('',(-23.5,-18.75,48.25));
#43798=CARTESIAN_POINT('Origin',(-18.75,-18.75,48.5));
#43799=CARTESIAN_POINT('Origin',(-18.75,-18.75,57.));
#43800=CARTESIAN_POINT('',(-23.25,-18.75,43.25));
#43801=CARTESIAN_POINT('',(-23.25,-18.75,57.));
#43802=CARTESIAN_POINT('Origin',(-18.75,-18.75,43.25));
#43803=CARTESIAN_POINT('Origin',(-18.75,-18.75,48.5));
#43804=CARTESIAN_POINT('',(-25.75,-18.75,48.5));
#43805=CARTESIAN_POINT('Origin',(-18.75,-18.75,48.5));
#43806=CARTESIAN_POINT('Origin',(18.75,-56.25,48.25));
#43807=CARTESIAN_POINT('',(14.25,-56.25,48.));
#43808=CARTESIAN_POINT('Origin',(18.75,-56.25,48.));
#43809=CARTESIAN_POINT('',(13.75,-56.25,48.5));
#43810=CARTESIAN_POINT('',(14.,-56.25,48.25));
#43811=CARTESIAN_POINT('Origin',(18.75,-56.25,48.5));
#43812=CARTESIAN_POINT('Origin',(18.75,-56.25,57.));
#43813=CARTESIAN_POINT('',(14.25,-56.25,43.25));
#43814=CARTESIAN_POINT('',(14.25,-56.25,57.));
#43815=CARTESIAN_POINT('Origin',(18.75,-56.25,43.25));
#43816=CARTESIAN_POINT('Origin',(18.75,-56.25,48.5));
#43817=CARTESIAN_POINT('',(11.75,-56.25,48.5));
#43818=CARTESIAN_POINT('Origin',(18.75,-56.25,48.5));
#43819=CARTESIAN_POINT('Origin',(18.75,-18.75,48.25));
#43820=CARTESIAN_POINT('',(14.25,-18.75,48.));
#43821=CARTESIAN_POINT('Origin',(18.75,-18.75,48.));
#43822=CARTESIAN_POINT('',(13.75,-18.75,48.5));
#43823=CARTESIAN_POINT('',(14.,-18.75,48.25));
#43824=CARTESIAN_POINT('Origin',(18.75,-18.75,48.5));
#43825=CARTESIAN_POINT('Origin',(18.75,-18.75,57.));
#43826=CARTESIAN_POINT('',(14.25,-18.75,43.25));
#43827=CARTESIAN_POINT('',(14.25,-18.75,57.));
#43828=CARTESIAN_POINT('Origin',(18.75,-18.75,43.25));
#43829=CARTESIAN_POINT('Origin',(18.75,-18.75,48.5));
#43830=CARTESIAN_POINT('',(11.75,-18.75,48.5));
#43831=CARTESIAN_POINT('Origin',(18.75,-18.75,48.5));
#43832=CARTESIAN_POINT('Origin',(56.25,-18.75,48.25));
#43833=CARTESIAN_POINT('',(51.75,-18.75,48.));
#43834=CARTESIAN_POINT('Origin',(56.25,-18.75,48.));
#43835=CARTESIAN_POINT('',(51.25,-18.75,48.5));
#43836=CARTESIAN_POINT('',(51.5,-18.75,48.25));
#43837=CARTESIAN_POINT('Origin',(56.25,-18.75,48.5));
#43838=CARTESIAN_POINT('Origin',(56.25,-18.75,57.));
#43839=CARTESIAN_POINT('',(51.75,-18.75,43.25));
#43840=CARTESIAN_POINT('',(51.75,-18.75,57.));
#43841=CARTESIAN_POINT('Origin',(56.25,-18.75,43.25));
#43842=CARTESIAN_POINT('Origin',(56.25,-18.75,48.5));
#43843=CARTESIAN_POINT('',(49.25,-18.75,48.5));
#43844=CARTESIAN_POINT('Origin',(56.25,-18.75,48.5));
#43845=CARTESIAN_POINT('Origin',(-52.425,52.425,47.));
#43846=CARTESIAN_POINT('',(-54.425,52.425,47.25));
#43847=CARTESIAN_POINT('Origin',(-52.425,52.425,47.25));
#43848=CARTESIAN_POINT('',(-54.925,52.425,46.75));
#43849=CARTESIAN_POINT('',(-54.675,52.425,47.));
#43850=CARTESIAN_POINT('Origin',(-52.425,52.425,46.75));
#43851=CARTESIAN_POINT('Origin',(-52.425,52.425,57.));
#43852=CARTESIAN_POINT('',(-54.425,52.425,56.5));
#43853=CARTESIAN_POINT('Origin',(-52.425,52.425,56.5));
#43854=CARTESIAN_POINT('',(-54.425,52.425,57.));
#43855=CARTESIAN_POINT('Origin',(-52.425,52.425,46.75));
#43856=CARTESIAN_POINT('',(-56.6629,52.425,46.75));
#43857=CARTESIAN_POINT('Origin',(-52.425,52.425,46.75));
#43858=CARTESIAN_POINT('Origin',(85.475,-85.475,42.75));
#43859=CARTESIAN_POINT('',(85.475,-85.475,56.75));
#43860=CARTESIAN_POINT('',(85.225,-85.725,56.5));
#43861=CARTESIAN_POINT('',(61.7520833333331,-109.197916666667,33.0270833333335));
#43862=CARTESIAN_POINT('',(85.225,-85.725,43.25));
#43863=CARTESIAN_POINT('',(85.225,-85.725,42.75));
#43864=CARTESIAN_POINT('',(85.475,-85.475,43.));
#43865=CARTESIAN_POINT('',(64.1270833333331,-106.822916666667,64.3479166666665));
#43866=CARTESIAN_POINT('',(85.725,-85.225,43.25));
#43867=CARTESIAN_POINT('',(92.5354166666667,-78.4145833333332,50.0604166666666));
#43868=CARTESIAN_POINT('',(85.725,-85.225,56.5));
#43869=CARTESIAN_POINT('',(85.725,-85.225,42.75));
#43870=CARTESIAN_POINT('',(94.9104166666667,-76.0395833333332,47.3145833333334));
#43871=CARTESIAN_POINT('Origin',(85.475,-42.8625,56.75));
#43872=CARTESIAN_POINT('',(85.725,85.225,56.5));
#43873=CARTESIAN_POINT('',(85.725,-42.8625,56.5));
#43874=CARTESIAN_POINT('',(85.475,85.475,56.75));
#43875=CARTESIAN_POINT('',(109.197916666667,61.7520833333331,33.0270833333335));
#43876=CARTESIAN_POINT('',(85.225,85.225,57.));
#43877=CARTESIAN_POINT('',(85.225,85.225,57.));
#43878=CARTESIAN_POINT('',(85.225,-85.225,57.));
#43879=CARTESIAN_POINT('',(85.225,-42.8625,57.));
#43880=CARTESIAN_POINT('',(85.225,-85.225,57.));
#43881=CARTESIAN_POINT('Origin',(85.725,-85.725,42.75));
#43882=CARTESIAN_POINT('',(85.725,85.225,43.25));
#43883=CARTESIAN_POINT('',(85.725,-42.8625,43.25));
#43884=CARTESIAN_POINT('',(85.725,85.225,42.75));
#43885=CARTESIAN_POINT('Origin',(85.475,-42.8625,43.));
#43886=CARTESIAN_POINT('',(85.225,-85.225,42.75));
#43887=CARTESIAN_POINT('',(85.225,-85.225,42.75));
#43888=CARTESIAN_POINT('',(85.225,85.225,42.75));
#43889=CARTESIAN_POINT('',(85.225,-42.8625,42.75));
#43890=CARTESIAN_POINT('',(85.475,85.475,43.));
#43891=CARTESIAN_POINT('',(85.225,85.225,42.75));
#43892=CARTESIAN_POINT('',(106.822916666667,64.1270833333331,64.3479166666665));
#43893=CARTESIAN_POINT('Origin',(-18.75,56.25,45.75));
#43894=CARTESIAN_POINT('',(-22.25,56.25,45.5));
#43895=CARTESIAN_POINT('Origin',(-18.75,56.25,45.5));
#43896=CARTESIAN_POINT('',(-22.75,56.25,46.));
#43897=CARTESIAN_POINT('',(-22.5,56.25,45.75));
#43898=CARTESIAN_POINT('Origin',(-18.75,56.25,46.));
#43899=CARTESIAN_POINT('Origin',(-18.75,56.25,57.));
#43900=CARTESIAN_POINT('',(-22.25,56.25,43.25));
#43901=CARTESIAN_POINT('',(-22.25,56.25,57.));
#43902=CARTESIAN_POINT('Origin',(-18.75,56.25,43.25));
#43903=CARTESIAN_POINT('Origin',(-18.75,56.25,46.));
#43904=CARTESIAN_POINT('',(-25.25,56.25,46.));
#43905=CARTESIAN_POINT('Origin',(-18.75,56.25,46.));
#43906=CARTESIAN_POINT('Origin',(-56.25,18.75,45.75));
#43907=CARTESIAN_POINT('',(-59.75,18.75,45.5));
#43908=CARTESIAN_POINT('Origin',(-56.25,18.75,45.5));
#43909=CARTESIAN_POINT('',(-60.25,18.75,46.));
#43910=CARTESIAN_POINT('',(-60.,18.75,45.75));
#43911=CARTESIAN_POINT('Origin',(-56.25,18.75,46.));
#43912=CARTESIAN_POINT('Origin',(-56.25,18.75,57.));
#43913=CARTESIAN_POINT('',(-59.75,18.75,43.25));
#43914=CARTESIAN_POINT('',(-59.75,18.75,57.));
#43915=CARTESIAN_POINT('Origin',(-56.25,18.75,43.25));
#43916=CARTESIAN_POINT('Origin',(-56.25,18.75,46.));
#43917=CARTESIAN_POINT('',(-62.75,18.75,46.));
#43918=CARTESIAN_POINT('Origin',(-56.25,18.75,46.));
#43919=CARTESIAN_POINT('Origin',(-85.475,-85.475,42.75));
#43920=CARTESIAN_POINT('',(-85.475,-85.475,56.75));
#43921=CARTESIAN_POINT('',(-85.725,-85.225,56.5));
#43922=CARTESIAN_POINT('',(-109.197916666667,-61.7520833333331,33.0270833333335));
#43923=CARTESIAN_POINT('',(-85.725,-85.225,43.25));
#43924=CARTESIAN_POINT('',(-85.725,-85.225,42.75));
#43925=CARTESIAN_POINT('',(-85.475,-85.475,43.));
#43926=CARTESIAN_POINT('',(-106.822916666667,-64.1270833333331,64.3479166666665));
#43927=CARTESIAN_POINT('',(-85.225,-85.725,43.25));
#43928=CARTESIAN_POINT('',(-78.4145833333332,-92.5354166666667,50.0604166666666));
#43929=CARTESIAN_POINT('',(-85.225,-85.725,56.5));
#43930=CARTESIAN_POINT('',(-85.225,-85.725,42.75));
#43931=CARTESIAN_POINT('',(-76.0395833333332,-94.9104166666667,47.3145833333334));
#43932=CARTESIAN_POINT('Origin',(-85.475,42.8625,43.));
#43933=CARTESIAN_POINT('',(-85.725,85.225,43.25));
#43934=CARTESIAN_POINT('',(-85.725,42.8625,43.25));
#43935=CARTESIAN_POINT('',(-85.475,85.475,43.));
#43936=CARTESIAN_POINT('',(-92.5354166666667,78.4145833333332,50.0604166666666));
#43937=CARTESIAN_POINT('',(-85.225,85.225,42.75));
#43938=CARTESIAN_POINT('',(-85.725,85.725,43.25));
#43939=CARTESIAN_POINT('',(-85.225,-85.225,42.75));
#43940=CARTESIAN_POINT('',(-85.225,42.8625,42.75));
#43941=CARTESIAN_POINT('',(-85.225,-85.225,42.75));
#43942=CARTESIAN_POINT('Origin',(-85.725,85.725,42.75));
#43943=CARTESIAN_POINT('',(-85.725,85.225,56.5));
#43944=CARTESIAN_POINT('',(-85.725,42.8625,56.5));
#43945=CARTESIAN_POINT('',(-85.725,85.225,42.75));
#43946=CARTESIAN_POINT('Origin',(-85.475,42.8625,56.75));
#43947=CARTESIAN_POINT('',(-85.225,-85.225,57.));
#43948=CARTESIAN_POINT('',(-85.225,-85.225,57.));
#43949=CARTESIAN_POINT('',(-85.225,85.225,57.));
#43950=CARTESIAN_POINT('',(-85.225,42.8625,57.));
#43951=CARTESIAN_POINT('',(-85.475,85.475,56.75));
#43952=CARTESIAN_POINT('',(-85.225,85.225,57.));
#43953=CARTESIAN_POINT('',(-94.9104166666667,76.0395833333332,47.3145833333334));
#43954=CARTESIAN_POINT('Origin',(85.475,85.475,42.75));
#43955=CARTESIAN_POINT('',(85.225,85.725,43.25));
#43956=CARTESIAN_POINT('',(78.4145833333332,92.5354166666667,50.0604166666666));
#43957=CARTESIAN_POINT('',(85.225,85.725,56.5));
#43958=CARTESIAN_POINT('',(85.225,85.725,42.75));
#43959=CARTESIAN_POINT('',(76.0395833333332,94.9104166666667,47.3145833333334));
#43960=CARTESIAN_POINT('Origin',(-85.475,85.475,42.75));
#43961=CARTESIAN_POINT('',(-85.225,85.725,56.5));
#43962=CARTESIAN_POINT('',(-61.7520833333331,109.197916666667,33.0270833333335));
#43963=CARTESIAN_POINT('',(-85.225,85.725,43.25));
#43964=CARTESIAN_POINT('',(-85.225,85.725,42.75));
#43965=CARTESIAN_POINT('',(-64.1270833333331,106.822916666667,64.3479166666665));
#43966=CARTESIAN_POINT('Origin',(56.25,18.75,48.25));
#43967=CARTESIAN_POINT('',(51.75,18.75,48.));
#43968=CARTESIAN_POINT('Origin',(56.25,18.75,48.));
#43969=CARTESIAN_POINT('',(51.25,18.75,48.5));
#43970=CARTESIAN_POINT('',(51.5,18.75,48.25));
#43971=CARTESIAN_POINT('Origin',(56.25,18.75,48.5));
#43972=CARTESIAN_POINT('Origin',(56.25,18.75,57.));
#43973=CARTESIAN_POINT('',(51.75,18.75,43.25));
#43974=CARTESIAN_POINT('',(51.75,18.75,57.));
#43975=CARTESIAN_POINT('Origin',(56.25,18.75,43.25));
#43976=CARTESIAN_POINT('Origin',(56.25,18.75,48.5));
#43977=CARTESIAN_POINT('',(49.25,18.75,48.5));
#43978=CARTESIAN_POINT('Origin',(56.25,18.75,48.5));
#43979=CARTESIAN_POINT('Origin',(18.75,56.25,48.25));
#43980=CARTESIAN_POINT('',(14.25,56.25,48.));
#43981=CARTESIAN_POINT('Origin',(18.75,56.25,48.));
#43982=CARTESIAN_POINT('',(13.75,56.25,48.5));
#43983=CARTESIAN_POINT('',(14.,56.25,48.25));
#43984=CARTESIAN_POINT('Origin',(18.75,56.25,48.5));
#43985=CARTESIAN_POINT('Origin',(18.75,56.25,57.));
#43986=CARTESIAN_POINT('',(14.25,56.25,43.25));
#43987=CARTESIAN_POINT('',(14.25,56.25,57.));
#43988=CARTESIAN_POINT('Origin',(18.75,56.25,43.25));
#43989=CARTESIAN_POINT('Origin',(18.75,56.25,48.5));
#43990=CARTESIAN_POINT('',(11.75,56.25,48.5));
#43991=CARTESIAN_POINT('Origin',(18.75,56.25,48.5));
#43992=CARTESIAN_POINT('Origin',(18.75,-18.75,43.));
#43993=CARTESIAN_POINT('',(13.75,-18.75,42.75));
#43994=CARTESIAN_POINT('Origin',(18.75,-18.75,42.75));
#43995=CARTESIAN_POINT('',(14.,-18.75,43.));
#43996=CARTESIAN_POINT('Origin',(0.,0.,42.75));
#43997=CARTESIAN_POINT('',(42.8625,85.225,42.75));
#43998=CARTESIAN_POINT('',(-42.8625,-85.225,42.75));
#43999=CARTESIAN_POINT('',(13.75,-56.25,42.75));
#44000=CARTESIAN_POINT('Origin',(18.75,-56.25,42.75));
#44001=CARTESIAN_POINT('',(-23.75,-56.25,42.75));
#44002=CARTESIAN_POINT('Origin',(-18.75,-56.25,42.75));
#44003=CARTESIAN_POINT('',(-61.25,-18.75,42.75));
#44004=CARTESIAN_POINT('Origin',(-56.25,-18.75,42.75));
#44005=CARTESIAN_POINT('',(51.25,-18.75,42.75));
#44006=CARTESIAN_POINT('Origin',(56.25,-18.75,42.75));
#44007=CARTESIAN_POINT('',(-59.975,-52.425,42.75));
#44008=CARTESIAN_POINT('Origin',(-52.425,-52.425,42.75));
#44009=CARTESIAN_POINT('',(51.25,18.75,42.75));
#44010=CARTESIAN_POINT('Origin',(56.25,18.75,42.75));
#44011=CARTESIAN_POINT('',(-42.05,56.25,42.75));
#44012=CARTESIAN_POINT('Origin',(-37.5,56.25,42.75));
#44013=CARTESIAN_POINT('',(-60.8,37.5,42.75));
#44014=CARTESIAN_POINT('Origin',(-56.25,37.5,42.75));
#44015=CARTESIAN_POINT('',(-23.3,-37.5,42.75));
#44016=CARTESIAN_POINT('Origin',(-18.75,-37.5,42.75));
#44017=CARTESIAN_POINT('',(-4.55,-18.75,42.75));
#44018=CARTESIAN_POINT('Origin',(0.,-18.75,42.75));
#44019=CARTESIAN_POINT('',(14.2,-37.5,42.75));
#44020=CARTESIAN_POINT('Origin',(18.75,-37.5,42.75));
#44021=CARTESIAN_POINT('',(32.95,-18.75,42.75));
#44022=CARTESIAN_POINT('Origin',(37.5,-18.75,42.75));
#44023=CARTESIAN_POINT('',(-60.25,18.75,42.75));
#44024=CARTESIAN_POINT('Origin',(-56.25,18.75,42.75));
#44025=CARTESIAN_POINT('',(-23.3,5.57214293612046E-16,42.75));
#44026=CARTESIAN_POINT('Origin',(-18.75,0.,42.75));
#44027=CARTESIAN_POINT('',(-60.8,5.57214293612046E-16,42.75));
#44028=CARTESIAN_POINT('Origin',(-56.25,0.,42.75));
#44029=CARTESIAN_POINT('',(14.2,5.57214293612045E-16,42.75));
#44030=CARTESIAN_POINT('Origin',(18.75,0.,42.75));
#44031=CARTESIAN_POINT('',(32.95,18.75,42.75));
#44032=CARTESIAN_POINT('Origin',(37.5,18.75,42.75));
#44033=CARTESIAN_POINT('',(29.5,-37.5,42.75));
#44034=CARTESIAN_POINT('Origin',(37.5,-37.5,42.75));
#44035=CARTESIAN_POINT('',(-8.,-37.5,42.75));
#44036=CARTESIAN_POINT('Origin',(0.,-37.5,42.75));
#44037=CARTESIAN_POINT('',(-8.,9.79717439317883E-16,42.75));
#44038=CARTESIAN_POINT('Origin',(0.,0.,42.75));
#44039=CARTESIAN_POINT('',(29.5,9.79717439317882E-16,42.75));
#44040=CARTESIAN_POINT('Origin',(37.5,0.,42.75));
#44041=CARTESIAN_POINT('',(-56.6629,52.425,42.75));
#44042=CARTESIAN_POINT('Origin',(-52.425,52.425,42.75));
#44043=CARTESIAN_POINT('',(-8.,37.5,42.75));
#44044=CARTESIAN_POINT('Origin',(0.,37.5,42.75));
#44045=CARTESIAN_POINT('',(-45.5,37.5,42.75));
#44046=CARTESIAN_POINT('Origin',(-37.5,37.5,42.75));
#44047=CARTESIAN_POINT('',(-45.5,9.79717439317882E-16,42.75));
#44048=CARTESIAN_POINT('Origin',(-37.5,0.,42.75));
#44049=CARTESIAN_POINT('',(51.7,5.57214293612046E-16,42.75));
#44050=CARTESIAN_POINT('Origin',(56.25,0.,42.75));
#44051=CARTESIAN_POINT('',(32.95,-56.25,42.75));
#44052=CARTESIAN_POINT('Origin',(37.5,-56.25,42.75));
#44053=CARTESIAN_POINT('',(-4.55,56.25,42.75));
#44054=CARTESIAN_POINT('Origin',(0.,56.25,42.75));
#44055=CARTESIAN_POINT('',(-4.55,-56.25,42.75));
#44056=CARTESIAN_POINT('Origin',(0.,-56.25,42.75));
#44057=CARTESIAN_POINT('',(-22.75,56.25,42.75));
#44058=CARTESIAN_POINT('Origin',(-18.75,56.25,42.75));
#44059=CARTESIAN_POINT('',(51.7,-37.5,42.75));
#44060=CARTESIAN_POINT('Origin',(56.25,-37.5,42.75));
#44061=CARTESIAN_POINT('',(14.2,37.5,42.75));
#44062=CARTESIAN_POINT('Origin',(18.75,37.5,42.75));
#44063=CARTESIAN_POINT('',(-4.55,18.75,42.75));
#44064=CARTESIAN_POINT('Origin',(0.,18.75,42.75));
#44065=CARTESIAN_POINT('',(-23.3,37.5,42.75));
#44066=CARTESIAN_POINT('Origin',(-18.75,37.5,42.75));
#44067=CARTESIAN_POINT('',(-42.05,18.75,42.75));
#44068=CARTESIAN_POINT('Origin',(-37.5,18.75,42.75));
#44069=CARTESIAN_POINT('',(-42.05,-18.75,42.75));
#44070=CARTESIAN_POINT('Origin',(-37.5,-18.75,42.75));
#44071=CARTESIAN_POINT('',(13.75,56.25,42.75));
#44072=CARTESIAN_POINT('Origin',(18.75,56.25,42.75));
#44073=CARTESIAN_POINT('',(44.875,52.425,42.75));
#44074=CARTESIAN_POINT('Origin',(52.425,52.425,42.75));
#44075=CARTESIAN_POINT('',(13.75,18.75,42.75));
#44076=CARTESIAN_POINT('Origin',(18.75,18.75,42.75));
#44077=CARTESIAN_POINT('',(-23.75,18.75,42.75));
#44078=CARTESIAN_POINT('Origin',(-18.75,18.75,42.75));
#44079=CARTESIAN_POINT('',(-23.75,-18.75,42.75));
#44080=CARTESIAN_POINT('Origin',(-18.75,-18.75,42.75));
#44081=CARTESIAN_POINT('Origin',(18.75,-56.25,43.));
#44082=CARTESIAN_POINT('',(14.,-56.25,43.));
#44083=CARTESIAN_POINT('Origin',(-18.75,-18.75,43.));
#44084=CARTESIAN_POINT('',(-23.5,-18.75,43.));
#44085=CARTESIAN_POINT('Origin',(-18.75,-56.25,43.));
#44086=CARTESIAN_POINT('',(-23.5,-56.25,43.));
#44087=CARTESIAN_POINT('Origin',(-18.75,18.75,43.));
#44088=CARTESIAN_POINT('',(-23.5,18.75,43.));
#44089=CARTESIAN_POINT('Origin',(-56.25,-18.75,43.));
#44090=CARTESIAN_POINT('',(-61.,-18.75,43.));
#44091=CARTESIAN_POINT('Origin',(18.75,18.75,43.));
#44092=CARTESIAN_POINT('',(14.,18.75,43.));
#44093=CARTESIAN_POINT('Origin',(56.25,-18.75,43.));
#44094=CARTESIAN_POINT('',(51.5,-18.75,43.));
#44095=CARTESIAN_POINT('Origin',(52.425,52.425,43.));
#44096=CARTESIAN_POINT('',(45.375,52.425,43.25));
#44097=CARTESIAN_POINT('',(45.125,52.425,43.));
#44098=CARTESIAN_POINT('Origin',(52.425,52.425,43.25));
#44099=CARTESIAN_POINT('Origin',(52.425,52.425,57.));
#44100=CARTESIAN_POINT('',(45.375,52.425,56.5));
#44101=CARTESIAN_POINT('Origin',(52.425,52.425,56.5));
#44102=CARTESIAN_POINT('',(45.375,52.425,57.));
#44103=CARTESIAN_POINT('Origin',(-52.425,-52.425,43.));
#44104=CARTESIAN_POINT('',(-59.475,-52.425,43.25));
#44105=CARTESIAN_POINT('',(-59.725,-52.425,43.));
#44106=CARTESIAN_POINT('Origin',(-52.425,-52.425,43.25));
#44107=CARTESIAN_POINT('Origin',(-52.425,-52.425,57.));
#44108=CARTESIAN_POINT('',(-59.475,-52.425,56.5));
#44109=CARTESIAN_POINT('Origin',(-52.425,-52.425,56.5));
#44110=CARTESIAN_POINT('',(-59.475,-52.425,57.));
#44111=CARTESIAN_POINT('Origin',(18.75,56.25,43.));
#44112=CARTESIAN_POINT('',(14.,56.25,43.));
#44113=CARTESIAN_POINT('Origin',(56.25,18.75,43.));
#44114=CARTESIAN_POINT('',(51.5,18.75,43.));
#44115=CARTESIAN_POINT('Origin',(42.8625,85.475,43.));
#44116=CARTESIAN_POINT('',(42.8625,85.725,43.25));
#44117=CARTESIAN_POINT('Origin',(-42.8625,-85.475,43.));
#44118=CARTESIAN_POINT('',(-42.8625,-85.725,43.25));
#44119=CARTESIAN_POINT('Origin',(85.725,85.725,42.75));
#44120=CARTESIAN_POINT('',(42.8625,85.725,56.5));
#44121=CARTESIAN_POINT('Origin',(-37.5,56.25,43.));
#44122=CARTESIAN_POINT('',(-41.55,56.25,43.25));
#44123=CARTESIAN_POINT('',(-41.8,56.25,43.));
#44124=CARTESIAN_POINT('Origin',(-37.5,56.25,43.25));
#44125=CARTESIAN_POINT('Origin',(-37.5,56.25,57.));
#44126=CARTESIAN_POINT('',(-41.55,56.25,56.5));
#44127=CARTESIAN_POINT('Origin',(-37.5,56.25,56.5));
#44128=CARTESIAN_POINT('',(-41.55,56.25,57.));
#44129=CARTESIAN_POINT('Origin',(-37.5,-18.75,43.));
#44130=CARTESIAN_POINT('',(-41.55,-18.75,43.25));
#44131=CARTESIAN_POINT('',(-41.8,-18.75,43.));
#44132=CARTESIAN_POINT('Origin',(-37.5,-18.75,43.25));
#44133=CARTESIAN_POINT('Origin',(-37.5,-18.75,57.));
#44134=CARTESIAN_POINT('',(-41.55,-18.75,56.5));
#44135=CARTESIAN_POINT('Origin',(-37.5,-18.75,56.5));
#44136=CARTESIAN_POINT('',(-41.55,-18.75,57.));
#44137=CARTESIAN_POINT('Origin',(-56.25,37.5,43.));
#44138=CARTESIAN_POINT('',(-60.3,37.5,43.25));
#44139=CARTESIAN_POINT('',(-60.55,37.5,43.));
#44140=CARTESIAN_POINT('Origin',(-56.25,37.5,43.25));
#44141=CARTESIAN_POINT('Origin',(-56.25,37.5,57.));
#44142=CARTESIAN_POINT('',(-60.3,37.5,56.5));
#44143=CARTESIAN_POINT('Origin',(-56.25,37.5,56.5));
#44144=CARTESIAN_POINT('',(-60.3,37.5,57.));
#44145=CARTESIAN_POINT('Origin',(-37.5,18.75,43.));
#44146=CARTESIAN_POINT('',(-41.55,18.75,43.25));
#44147=CARTESIAN_POINT('',(-41.8,18.75,43.));
#44148=CARTESIAN_POINT('Origin',(-37.5,18.75,43.25));
#44149=CARTESIAN_POINT('Origin',(-37.5,18.75,57.));
#44150=CARTESIAN_POINT('',(-41.55,18.75,56.5));
#44151=CARTESIAN_POINT('Origin',(-37.5,18.75,56.5));
#44152=CARTESIAN_POINT('',(-41.55,18.75,57.));
#44153=CARTESIAN_POINT('Origin',(-18.75,-37.5,43.));
#44154=CARTESIAN_POINT('',(-22.8,-37.5,43.25));
#44155=CARTESIAN_POINT('',(-23.05,-37.5,43.));
#44156=CARTESIAN_POINT('Origin',(-18.75,-37.5,43.25));
#44157=CARTESIAN_POINT('Origin',(-18.75,-37.5,57.));
#44158=CARTESIAN_POINT('',(-22.8,-37.5,56.5));
#44159=CARTESIAN_POINT('Origin',(-18.75,-37.5,56.5));
#44160=CARTESIAN_POINT('',(-22.8,-37.5,57.));
#44161=CARTESIAN_POINT('Origin',(-18.75,37.5,43.));
#44162=CARTESIAN_POINT('',(-22.8,37.5,43.25));
#44163=CARTESIAN_POINT('',(-23.05,37.5,43.));
#44164=CARTESIAN_POINT('Origin',(-18.75,37.5,43.25));
#44165=CARTESIAN_POINT('Origin',(-18.75,37.5,57.));
#44166=CARTESIAN_POINT('',(-22.8,37.5,56.5));
#44167=CARTESIAN_POINT('Origin',(-18.75,37.5,56.5));
#44168=CARTESIAN_POINT('',(-22.8,37.5,57.));
#44169=CARTESIAN_POINT('Origin',(0.,-18.75,43.));
#44170=CARTESIAN_POINT('',(-4.05,-18.75,43.25));
#44171=CARTESIAN_POINT('',(-4.3,-18.75,43.));
#44172=CARTESIAN_POINT('Origin',(0.,-18.75,43.25));
#44173=CARTESIAN_POINT('Origin',(0.,-18.75,57.));
#44174=CARTESIAN_POINT('',(-4.05,-18.75,56.5));
#44175=CARTESIAN_POINT('Origin',(0.,-18.75,56.5));
#44176=CARTESIAN_POINT('',(-4.05,-18.75,57.));
#44177=CARTESIAN_POINT('Origin',(0.,18.75,43.));
#44178=CARTESIAN_POINT('',(-4.05,18.75,43.25));
#44179=CARTESIAN_POINT('',(-4.3,18.75,43.));
#44180=CARTESIAN_POINT('Origin',(0.,18.75,43.25));
#44181=CARTESIAN_POINT('Origin',(0.,18.75,57.));
#44182=CARTESIAN_POINT('',(-4.05,18.75,56.5));
#44183=CARTESIAN_POINT('Origin',(0.,18.75,56.5));
#44184=CARTESIAN_POINT('',(-4.05,18.75,57.));
#44185=CARTESIAN_POINT('Origin',(18.75,-37.5,43.));
#44186=CARTESIAN_POINT('',(14.7,-37.5,43.25));
#44187=CARTESIAN_POINT('',(14.45,-37.5,43.));
#44188=CARTESIAN_POINT('Origin',(18.75,-37.5,43.25));
#44189=CARTESIAN_POINT('Origin',(18.75,-37.5,57.));
#44190=CARTESIAN_POINT('',(14.7,-37.5,56.5));
#44191=CARTESIAN_POINT('Origin',(18.75,-37.5,56.5));
#44192=CARTESIAN_POINT('',(14.7,-37.5,57.));
#44193=CARTESIAN_POINT('Origin',(18.75,37.5,43.));
#44194=CARTESIAN_POINT('',(14.7,37.5,43.25));
#44195=CARTESIAN_POINT('',(14.45,37.5,43.));
#44196=CARTESIAN_POINT('Origin',(18.75,37.5,43.25));
#44197=CARTESIAN_POINT('Origin',(18.75,37.5,57.));
#44198=CARTESIAN_POINT('',(14.7,37.5,56.5));
#44199=CARTESIAN_POINT('Origin',(18.75,37.5,56.5));
#44200=CARTESIAN_POINT('',(14.7,37.5,57.));
#44201=CARTESIAN_POINT('Origin',(37.5,-18.75,43.));
#44202=CARTESIAN_POINT('',(33.45,-18.75,43.25));
#44203=CARTESIAN_POINT('',(33.2,-18.75,43.));
#44204=CARTESIAN_POINT('Origin',(37.5,-18.75,43.25));
#44205=CARTESIAN_POINT('Origin',(37.5,-18.75,57.));
#44206=CARTESIAN_POINT('',(33.45,-18.75,56.5));
#44207=CARTESIAN_POINT('Origin',(37.5,-18.75,56.5));
#44208=CARTESIAN_POINT('',(33.45,-18.75,57.));
#44209=CARTESIAN_POINT('Origin',(56.25,-37.5,43.));
#44210=CARTESIAN_POINT('',(52.2,-37.5,43.25));
#44211=CARTESIAN_POINT('',(51.95,-37.5,43.));
#44212=CARTESIAN_POINT('Origin',(56.25,-37.5,43.25));
#44213=CARTESIAN_POINT('Origin',(56.25,-37.5,57.));
#44214=CARTESIAN_POINT('',(52.2,-37.5,56.5));
#44215=CARTESIAN_POINT('Origin',(56.25,-37.5,56.5));
#44216=CARTESIAN_POINT('',(52.2,-37.5,57.));
#44217=CARTESIAN_POINT('Origin',(-56.25,18.75,43.));
#44218=CARTESIAN_POINT('',(-60.,18.75,43.));
#44219=CARTESIAN_POINT('Origin',(-18.75,56.25,43.));
#44220=CARTESIAN_POINT('',(-22.5,56.25,43.));
#44221=CARTESIAN_POINT('Origin',(-18.75,0.,43.));
#44222=CARTESIAN_POINT('',(-22.8,-4.95981953654678E-16,43.25));
#44223=CARTESIAN_POINT('',(-23.05,5.26598123633362E-16,43.));
#44224=CARTESIAN_POINT('Origin',(-18.75,0.,43.25));
#44225=CARTESIAN_POINT('Origin',(-18.75,0.,57.));
#44226=CARTESIAN_POINT('',(-22.8,4.95981953654678E-16,56.5));
#44227=CARTESIAN_POINT('Origin',(-18.75,0.,56.5));
#44228=CARTESIAN_POINT('',(-22.8,4.95981953654678E-16,57.));
#44229=CARTESIAN_POINT('Origin',(0.,-56.25,43.));
#44230=CARTESIAN_POINT('',(-4.05,-56.25,43.25));
#44231=CARTESIAN_POINT('',(-4.3,-56.25,43.));
#44232=CARTESIAN_POINT('Origin',(0.,-56.25,43.25));
#44233=CARTESIAN_POINT('Origin',(0.,-56.25,57.));
#44234=CARTESIAN_POINT('',(-4.05,-56.25,56.5));
#44235=CARTESIAN_POINT('Origin',(0.,-56.25,56.5));
#44236=CARTESIAN_POINT('',(-4.05,-56.25,57.));
#44237=CARTESIAN_POINT('Origin',(-56.25,0.,43.));
#44238=CARTESIAN_POINT('',(-60.3,-4.95981953654678E-16,43.25));
#44239=CARTESIAN_POINT('',(-60.55,5.26598123633362E-16,43.));
#44240=CARTESIAN_POINT('Origin',(-56.25,0.,43.25));
#44241=CARTESIAN_POINT('Origin',(-56.25,0.,57.));
#44242=CARTESIAN_POINT('',(-60.3,4.95981953654678E-16,56.5));
#44243=CARTESIAN_POINT('Origin',(-56.25,0.,56.5));
#44244=CARTESIAN_POINT('',(-60.3,4.95981953654678E-16,57.));
#44245=CARTESIAN_POINT('Origin',(0.,56.25,43.));
#44246=CARTESIAN_POINT('',(-4.05,56.25,43.25));
#44247=CARTESIAN_POINT('',(-4.3,56.25,43.));
#44248=CARTESIAN_POINT('Origin',(0.,56.25,43.25));
#44249=CARTESIAN_POINT('Origin',(0.,56.25,57.));
#44250=CARTESIAN_POINT('',(-4.05,56.25,56.5));
#44251=CARTESIAN_POINT('Origin',(0.,56.25,56.5));
#44252=CARTESIAN_POINT('',(-4.05,56.25,57.));
#44253=CARTESIAN_POINT('Origin',(18.75,0.,43.));
#44254=CARTESIAN_POINT('',(14.7,-4.95981953654678E-16,43.25));
#44255=CARTESIAN_POINT('',(14.45,5.26598123633362E-16,43.));
#44256=CARTESIAN_POINT('Origin',(18.75,0.,43.25));
#44257=CARTESIAN_POINT('Origin',(18.75,0.,57.));
#44258=CARTESIAN_POINT('',(14.7,4.95981953654678E-16,56.5));
#44259=CARTESIAN_POINT('Origin',(18.75,0.,56.5));
#44260=CARTESIAN_POINT('',(14.7,4.95981953654678E-16,57.));
#44261=CARTESIAN_POINT('Origin',(37.5,-56.25,43.));
#44262=CARTESIAN_POINT('',(33.45,-56.25,43.25));
#44263=CARTESIAN_POINT('',(33.2,-56.25,43.));
#44264=CARTESIAN_POINT('Origin',(37.5,-56.25,43.25));
#44265=CARTESIAN_POINT('Origin',(37.5,-56.25,57.));
#44266=CARTESIAN_POINT('',(33.45,-56.25,56.5));
#44267=CARTESIAN_POINT('Origin',(37.5,-56.25,56.5));
#44268=CARTESIAN_POINT('',(33.45,-56.25,57.));
#44269=CARTESIAN_POINT('Origin',(37.5,18.75,43.));
#44270=CARTESIAN_POINT('',(33.45,18.75,43.25));
#44271=CARTESIAN_POINT('',(33.2,18.75,43.));
#44272=CARTESIAN_POINT('Origin',(37.5,18.75,43.25));
#44273=CARTESIAN_POINT('Origin',(37.5,18.75,57.));
#44274=CARTESIAN_POINT('',(33.45,18.75,56.5));
#44275=CARTESIAN_POINT('Origin',(37.5,18.75,56.5));
#44276=CARTESIAN_POINT('',(33.45,18.75,57.));
#44277=CARTESIAN_POINT('Origin',(56.25,0.,43.));
#44278=CARTESIAN_POINT('',(52.2,-4.95981953654678E-16,43.25));
#44279=CARTESIAN_POINT('',(51.95,5.26598123633362E-16,43.));
#44280=CARTESIAN_POINT('Origin',(56.25,0.,43.25));
#44281=CARTESIAN_POINT('Origin',(56.25,0.,57.));
#44282=CARTESIAN_POINT('',(52.2,4.95981953654678E-16,56.5));
#44283=CARTESIAN_POINT('Origin',(56.25,0.,56.5));
#44284=CARTESIAN_POINT('',(52.2,4.95981953654678E-16,57.));
#44285=CARTESIAN_POINT('Origin',(37.5,-37.5,43.));
#44286=CARTESIAN_POINT('',(30.,-37.5,43.25));
#44287=CARTESIAN_POINT('',(29.75,-37.5,43.));
#44288=CARTESIAN_POINT('Origin',(37.5,-37.5,43.25));
#44289=CARTESIAN_POINT('Origin',(37.5,-37.5,57.));
#44290=CARTESIAN_POINT('',(30.,-37.5,56.5));
#44291=CARTESIAN_POINT('Origin',(37.5,-37.5,56.5));
#44292=CARTESIAN_POINT('',(30.,-37.5,57.));
#44293=CARTESIAN_POINT('Origin',(-37.5,0.,43.));
#44294=CARTESIAN_POINT('',(-45.,-9.18485099360515E-16,43.25));
#44295=CARTESIAN_POINT('',(-45.25,9.49101269339199E-16,43.));
#44296=CARTESIAN_POINT('Origin',(-37.5,0.,43.25));
#44297=CARTESIAN_POINT('Origin',(-37.5,0.,57.));
#44298=CARTESIAN_POINT('',(-45.,9.18485099360515E-16,56.5));
#44299=CARTESIAN_POINT('Origin',(-37.5,0.,56.5));
#44300=CARTESIAN_POINT('',(-45.,9.18485099360515E-16,57.));
#44301=CARTESIAN_POINT('Origin',(0.,-37.5,43.));
#44302=CARTESIAN_POINT('',(-7.5,-37.5,43.25));
#44303=CARTESIAN_POINT('',(-7.75,-37.5,43.));
#44304=CARTESIAN_POINT('Origin',(0.,-37.5,43.25));
#44305=CARTESIAN_POINT('Origin',(0.,-37.5,57.));
#44306=CARTESIAN_POINT('',(-7.5,-37.5,56.5));
#44307=CARTESIAN_POINT('Origin',(0.,-37.5,56.5));
#44308=CARTESIAN_POINT('',(-7.5,-37.5,57.));
#44309=CARTESIAN_POINT('Origin',(-37.5,37.5,43.));
#44310=CARTESIAN_POINT('',(-45.,37.5,43.25));
#44311=CARTESIAN_POINT('',(-45.25,37.5,43.));
#44312=CARTESIAN_POINT('Origin',(-37.5,37.5,43.25));
#44313=CARTESIAN_POINT('Origin',(-37.5,37.5,57.));
#44314=CARTESIAN_POINT('',(-45.,37.5,56.5));
#44315=CARTESIAN_POINT('Origin',(-37.5,37.5,56.5));
#44316=CARTESIAN_POINT('',(-45.,37.5,57.));
#44317=CARTESIAN_POINT('Origin',(0.,0.,43.));
#44318=CARTESIAN_POINT('',(-7.5,-9.18485099360515E-16,43.25));
#44319=CARTESIAN_POINT('',(-7.75,9.49101269339199E-16,43.));
#44320=CARTESIAN_POINT('Origin',(0.,0.,43.25));
#44321=CARTESIAN_POINT('Origin',(0.,0.,57.));
#44322=CARTESIAN_POINT('',(-7.5,9.18485099360515E-16,56.5));
#44323=CARTESIAN_POINT('Origin',(0.,0.,56.5));
#44324=CARTESIAN_POINT('',(-7.5,9.18485099360515E-16,57.));
#44325=CARTESIAN_POINT('Origin',(0.,37.5,43.));
#44326=CARTESIAN_POINT('',(-7.5,37.5,43.25));
#44327=CARTESIAN_POINT('',(-7.75,37.5,43.));
#44328=CARTESIAN_POINT('Origin',(0.,37.5,43.25));
#44329=CARTESIAN_POINT('Origin',(0.,37.5,57.));
#44330=CARTESIAN_POINT('',(-7.5,37.5,56.5));
#44331=CARTESIAN_POINT('Origin',(0.,37.5,56.5));
#44332=CARTESIAN_POINT('',(-7.5,37.5,57.));
#44333=CARTESIAN_POINT('Origin',(37.5,0.,43.));
#44334=CARTESIAN_POINT('',(30.,-9.18485099360515E-16,43.25));
#44335=CARTESIAN_POINT('',(29.75,9.49101269339199E-16,43.));
#44336=CARTESIAN_POINT('Origin',(37.5,0.,43.25));
#44337=CARTESIAN_POINT('Origin',(37.5,0.,57.));
#44338=CARTESIAN_POINT('',(30.,9.18485099360515E-16,56.5));
#44339=CARTESIAN_POINT('Origin',(37.5,0.,56.5));
#44340=CARTESIAN_POINT('',(30.,9.18485099360515E-16,57.));
#44341=CARTESIAN_POINT('Origin',(-42.8625,-85.475,56.75));
#44342=CARTESIAN_POINT('',(-42.8625,-85.225,57.));
#44343=CARTESIAN_POINT('',(-42.8625,-85.725,56.5));
#44344=CARTESIAN_POINT('Origin',(42.8625,85.475,56.75));
#44345=CARTESIAN_POINT('',(42.8625,85.225,57.));
#44346=CARTESIAN_POINT('Origin',(0.,0.,57.));
#44347=CARTESIAN_POINT('',(-54.925,52.425,57.));
#44348=CARTESIAN_POINT('Origin',(-52.425,52.425,57.));
#44349=CARTESIAN_POINT('',(-8.,37.5,57.));
#44350=CARTESIAN_POINT('Origin',(0.,37.5,57.));
#44351=CARTESIAN_POINT('',(-45.5,37.5,57.));
#44352=CARTESIAN_POINT('Origin',(-37.5,37.5,57.));
#44353=CARTESIAN_POINT('',(-45.5,-9.79717439317882E-16,57.));
#44354=CARTESIAN_POINT('Origin',(-37.5,0.,57.));
#44355=CARTESIAN_POINT('',(48.75,18.75,57.));
#44356=CARTESIAN_POINT('Origin',(56.25,18.75,57.));
#44357=CARTESIAN_POINT('',(11.25,-18.75,57.));
#44358=CARTESIAN_POINT('Origin',(18.75,-18.75,57.));
#44359=CARTESIAN_POINT('',(-26.25,-18.75,57.));
#44360=CARTESIAN_POINT('Origin',(-18.75,-18.75,57.));
#44361=CARTESIAN_POINT('',(-26.25,18.75,57.));
#44362=CARTESIAN_POINT('Origin',(-18.75,18.75,57.));
#44363=CARTESIAN_POINT('',(11.25,18.75,57.));
#44364=CARTESIAN_POINT('Origin',(18.75,18.75,57.));
#44365=CARTESIAN_POINT('',(51.7,-5.57214293612046E-16,57.));
#44366=CARTESIAN_POINT('Origin',(56.25,0.,57.));
#44367=CARTESIAN_POINT('',(32.95,-56.25,57.));
#44368=CARTESIAN_POINT('Origin',(37.5,-56.25,57.));
#44369=CARTESIAN_POINT('',(-4.55,56.25,57.));
#44370=CARTESIAN_POINT('Origin',(0.,56.25,57.));
#44371=CARTESIAN_POINT('',(-4.55,-56.25,57.));
#44372=CARTESIAN_POINT('Origin',(0.,-56.25,57.));
#44373=CARTESIAN_POINT('',(-42.05,56.25,57.));
#44374=CARTESIAN_POINT('Origin',(-37.5,56.25,57.));
#44375=CARTESIAN_POINT('',(-60.8,37.5,57.));
#44376=CARTESIAN_POINT('Origin',(-56.25,37.5,57.));
#44377=CARTESIAN_POINT('',(-23.3,-37.5,57.));
#44378=CARTESIAN_POINT('Origin',(-18.75,-37.5,57.));
#44379=CARTESIAN_POINT('',(-4.55,-18.75,57.));
#44380=CARTESIAN_POINT('Origin',(0.,-18.75,57.));
#44381=CARTESIAN_POINT('',(14.2,-37.5,57.));
#44382=CARTESIAN_POINT('Origin',(18.75,-37.5,57.));
#44383=CARTESIAN_POINT('',(32.95,-18.75,57.));
#44384=CARTESIAN_POINT('Origin',(37.5,-18.75,57.));
#44385=CARTESIAN_POINT('',(44.875,52.425,57.));
#44386=CARTESIAN_POINT('Origin',(52.425,52.425,57.));
#44387=CARTESIAN_POINT('',(-63.25,18.75,57.));
#44388=CARTESIAN_POINT('Origin',(-56.25,18.75,57.));
#44389=CARTESIAN_POINT('',(-25.75,56.25,57.));
#44390=CARTESIAN_POINT('Origin',(-18.75,56.25,57.));
#44391=CARTESIAN_POINT('',(-59.975,-52.425,57.));
#44392=CARTESIAN_POINT('Origin',(-52.425,-52.425,57.));
#44393=CARTESIAN_POINT('',(51.7,-37.5,57.));
#44394=CARTESIAN_POINT('Origin',(56.25,-37.5,57.));
#44395=CARTESIAN_POINT('',(14.2,37.5,57.));
#44396=CARTESIAN_POINT('Origin',(18.75,37.5,57.));
#44397=CARTESIAN_POINT('',(-4.55,18.75,57.));
#44398=CARTESIAN_POINT('Origin',(0.,18.75,57.));
#44399=CARTESIAN_POINT('',(-23.3,37.5,57.));
#44400=CARTESIAN_POINT('Origin',(-18.75,37.5,57.));
#44401=CARTESIAN_POINT('',(-42.05,18.75,57.));
#44402=CARTESIAN_POINT('Origin',(-37.5,18.75,57.));
#44403=CARTESIAN_POINT('',(-42.05,-18.75,57.));
#44404=CARTESIAN_POINT('Origin',(-37.5,-18.75,57.));
#44405=CARTESIAN_POINT('',(-23.3,-5.57214293612046E-16,57.));
#44406=CARTESIAN_POINT('Origin',(-18.75,0.,57.));
#44407=CARTESIAN_POINT('',(-60.8,-5.57214293612046E-16,57.));
#44408=CARTESIAN_POINT('Origin',(-56.25,0.,57.));
#44409=CARTESIAN_POINT('',(14.2,-5.57214293612045E-16,57.));
#44410=CARTESIAN_POINT('Origin',(18.75,0.,57.));
#44411=CARTESIAN_POINT('',(32.95,18.75,57.));
#44412=CARTESIAN_POINT('Origin',(37.5,18.75,57.));
#44413=CARTESIAN_POINT('',(48.75,-18.75,57.));
#44414=CARTESIAN_POINT('Origin',(56.25,-18.75,57.));
#44415=CARTESIAN_POINT('',(-63.75,-18.75,57.));
#44416=CARTESIAN_POINT('Origin',(-56.25,-18.75,57.));
#44417=CARTESIAN_POINT('',(-26.25,-56.25,57.));
#44418=CARTESIAN_POINT('Origin',(-18.75,-56.25,57.));
#44419=CARTESIAN_POINT('',(11.25,-56.25,57.));
#44420=CARTESIAN_POINT('Origin',(18.75,-56.25,57.));
#44421=CARTESIAN_POINT('',(11.25,56.25,57.));
#44422=CARTESIAN_POINT('Origin',(18.75,56.25,57.));
#44423=CARTESIAN_POINT('',(29.5,-37.5,57.));
#44424=CARTESIAN_POINT('Origin',(37.5,-37.5,57.));
#44425=CARTESIAN_POINT('',(-8.,-37.5,57.));
#44426=CARTESIAN_POINT('Origin',(0.,-37.5,57.));
#44427=CARTESIAN_POINT('',(-8.,-9.79717439317883E-16,57.));
#44428=CARTESIAN_POINT('Origin',(0.,0.,57.));
#44429=CARTESIAN_POINT('',(29.5,-9.79717439317882E-16,57.));
#44430=CARTESIAN_POINT('Origin',(37.5,0.,57.));
#44431=CARTESIAN_POINT('Origin',(-52.425,52.425,56.75));
#44432=CARTESIAN_POINT('',(-54.675,52.425,56.75));
#44433=CARTESIAN_POINT('Origin',(37.5,0.,56.75));
#44434=CARTESIAN_POINT('',(29.75,-9.49101269339199E-16,56.75));
#44435=CARTESIAN_POINT('Origin',(0.,37.5,56.75));
#44436=CARTESIAN_POINT('',(-7.75,37.5,56.75));
#44437=CARTESIAN_POINT('Origin',(0.,0.,56.75));
#44438=CARTESIAN_POINT('',(-7.75,-9.49101269339199E-16,56.75));
#44439=CARTESIAN_POINT('Origin',(-37.5,37.5,56.75));
#44440=CARTESIAN_POINT('',(-45.25,37.5,56.75));
#44441=CARTESIAN_POINT('Origin',(0.,-37.5,56.75));
#44442=CARTESIAN_POINT('',(-7.75,-37.5,56.75));
#44443=CARTESIAN_POINT('Origin',(-37.5,0.,56.75));
#44444=CARTESIAN_POINT('',(-45.25,-9.49101269339199E-16,56.75));
#44445=CARTESIAN_POINT('Origin',(37.5,-37.5,56.75));
#44446=CARTESIAN_POINT('',(29.75,-37.5,56.75));
#44447=CARTESIAN_POINT('Origin',(56.25,18.75,56.75));
#44448=CARTESIAN_POINT('',(49.25,18.75,56.5));
#44449=CARTESIAN_POINT('',(49.,18.75,56.75));
#44450=CARTESIAN_POINT('Origin',(56.25,18.75,56.5));
#44451=CARTESIAN_POINT('Origin',(56.25,18.75,57.));
#44452=CARTESIAN_POINT('',(49.25,18.75,57.));
#44453=CARTESIAN_POINT('Origin',(18.75,56.25,56.75));
#44454=CARTESIAN_POINT('',(11.75,56.25,56.5));
#44455=CARTESIAN_POINT('',(11.5,56.25,56.75));
#44456=CARTESIAN_POINT('Origin',(18.75,56.25,56.5));
#44457=CARTESIAN_POINT('Origin',(18.75,56.25,57.));
#44458=CARTESIAN_POINT('',(11.75,56.25,57.));
#44459=CARTESIAN_POINT('Origin',(18.75,-18.75,56.75));
#44460=CARTESIAN_POINT('',(11.75,-18.75,56.5));
#44461=CARTESIAN_POINT('',(11.5,-18.75,56.75));
#44462=CARTESIAN_POINT('Origin',(18.75,-18.75,56.5));
#44463=CARTESIAN_POINT('Origin',(18.75,-18.75,57.));
#44464=CARTESIAN_POINT('',(11.75,-18.75,57.));
#44465=CARTESIAN_POINT('Origin',(18.75,-56.25,56.75));
#44466=CARTESIAN_POINT('',(11.75,-56.25,56.5));
#44467=CARTESIAN_POINT('',(11.5,-56.25,56.75));
#44468=CARTESIAN_POINT('Origin',(18.75,-56.25,56.5));
#44469=CARTESIAN_POINT('Origin',(18.75,-56.25,57.));
#44470=CARTESIAN_POINT('',(11.75,-56.25,57.));
#44471=CARTESIAN_POINT('Origin',(-18.75,-18.75,56.75));
#44472=CARTESIAN_POINT('',(-25.75,-18.75,56.5));
#44473=CARTESIAN_POINT('',(-26.,-18.75,56.75));
#44474=CARTESIAN_POINT('Origin',(-18.75,-18.75,56.5));
#44475=CARTESIAN_POINT('Origin',(-18.75,-18.75,57.));
#44476=CARTESIAN_POINT('',(-25.75,-18.75,57.));
#44477=CARTESIAN_POINT('Origin',(-18.75,-56.25,56.75));
#44478=CARTESIAN_POINT('',(-25.75,-56.25,56.5));
#44479=CARTESIAN_POINT('',(-26.,-56.25,56.75));
#44480=CARTESIAN_POINT('Origin',(-18.75,-56.25,56.5));
#44481=CARTESIAN_POINT('Origin',(-18.75,-56.25,57.));
#44482=CARTESIAN_POINT('',(-25.75,-56.25,57.));
#44483=CARTESIAN_POINT('Origin',(-18.75,18.75,56.75));
#44484=CARTESIAN_POINT('',(-25.75,18.75,56.5));
#44485=CARTESIAN_POINT('',(-26.,18.75,56.75));
#44486=CARTESIAN_POINT('Origin',(-18.75,18.75,56.5));
#44487=CARTESIAN_POINT('Origin',(-18.75,18.75,57.));
#44488=CARTESIAN_POINT('',(-25.75,18.75,57.));
#44489=CARTESIAN_POINT('Origin',(-56.25,-18.75,56.75));
#44490=CARTESIAN_POINT('',(-63.25,-18.75,56.5));
#44491=CARTESIAN_POINT('',(-63.5,-18.75,56.75));
#44492=CARTESIAN_POINT('Origin',(-56.25,-18.75,56.5));
#44493=CARTESIAN_POINT('Origin',(-56.25,-18.75,57.));
#44494=CARTESIAN_POINT('',(-63.25,-18.75,57.));
#44495=CARTESIAN_POINT('Origin',(18.75,18.75,56.75));
#44496=CARTESIAN_POINT('',(11.75,18.75,56.5));
#44497=CARTESIAN_POINT('',(11.5,18.75,56.75));
#44498=CARTESIAN_POINT('Origin',(18.75,18.75,56.5));
#44499=CARTESIAN_POINT('Origin',(18.75,18.75,57.));
#44500=CARTESIAN_POINT('',(11.75,18.75,57.));
#44501=CARTESIAN_POINT('Origin',(56.25,-18.75,56.75));
#44502=CARTESIAN_POINT('',(49.25,-18.75,56.5));
#44503=CARTESIAN_POINT('',(49.,-18.75,56.75));
#44504=CARTESIAN_POINT('Origin',(56.25,-18.75,56.5));
#44505=CARTESIAN_POINT('Origin',(56.25,-18.75,57.));
#44506=CARTESIAN_POINT('',(49.25,-18.75,57.));
#44507=CARTESIAN_POINT('Origin',(56.25,0.,56.75));
#44508=CARTESIAN_POINT('',(51.95,-5.26598123633362E-16,56.75));
#44509=CARTESIAN_POINT('Origin',(37.5,18.75,56.75));
#44510=CARTESIAN_POINT('',(33.2,18.75,56.75));
#44511=CARTESIAN_POINT('Origin',(37.5,-56.25,56.75));
#44512=CARTESIAN_POINT('',(33.2,-56.25,56.75));
#44513=CARTESIAN_POINT('Origin',(18.75,0.,56.75));
#44514=CARTESIAN_POINT('',(14.45,-5.26598123633362E-16,56.75));
#44515=CARTESIAN_POINT('Origin',(0.,56.25,56.75));
#44516=CARTESIAN_POINT('',(-4.3,56.25,56.75));
#44517=CARTESIAN_POINT('Origin',(-56.25,0.,56.75));
#44518=CARTESIAN_POINT('',(-60.55,-5.26598123633362E-16,56.75));
#44519=CARTESIAN_POINT('Origin',(0.,-56.25,56.75));
#44520=CARTESIAN_POINT('',(-4.3,-56.25,56.75));
#44521=CARTESIAN_POINT('Origin',(-18.75,0.,56.75));
#44522=CARTESIAN_POINT('',(-23.05,-5.26598123633362E-16,56.75));
#44523=CARTESIAN_POINT('Origin',(-37.5,56.25,56.75));
#44524=CARTESIAN_POINT('',(-41.8,56.25,56.75));
#44525=CARTESIAN_POINT('Origin',(-37.5,-18.75,56.75));
#44526=CARTESIAN_POINT('',(-41.8,-18.75,56.75));
#44527=CARTESIAN_POINT('Origin',(-56.25,37.5,56.75));
#44528=CARTESIAN_POINT('',(-60.55,37.5,56.75));
#44529=CARTESIAN_POINT('Origin',(-37.5,18.75,56.75));
#44530=CARTESIAN_POINT('',(-41.8,18.75,56.75));
#44531=CARTESIAN_POINT('Origin',(-18.75,-37.5,56.75));
#44532=CARTESIAN_POINT('',(-23.05,-37.5,56.75));
#44533=CARTESIAN_POINT('Origin',(-18.75,37.5,56.75));
#44534=CARTESIAN_POINT('',(-23.05,37.5,56.75));
#44535=CARTESIAN_POINT('Origin',(0.,-18.75,56.75));
#44536=CARTESIAN_POINT('',(-4.3,-18.75,56.75));
#44537=CARTESIAN_POINT('Origin',(0.,18.75,56.75));
#44538=CARTESIAN_POINT('',(-4.3,18.75,56.75));
#44539=CARTESIAN_POINT('Origin',(18.75,-37.5,56.75));
#44540=CARTESIAN_POINT('',(14.45,-37.5,56.75));
#44541=CARTESIAN_POINT('Origin',(18.75,37.5,56.75));
#44542=CARTESIAN_POINT('',(14.45,37.5,56.75));
#44543=CARTESIAN_POINT('Origin',(37.5,-18.75,56.75));
#44544=CARTESIAN_POINT('',(33.2,-18.75,56.75));
#44545=CARTESIAN_POINT('Origin',(56.25,-37.5,56.75));
#44546=CARTESIAN_POINT('',(51.95,-37.5,56.75));
#44547=CARTESIAN_POINT('Origin',(52.425,52.425,56.75));
#44548=CARTESIAN_POINT('',(45.125,52.425,56.75));
#44549=CARTESIAN_POINT('Origin',(-52.425,-52.425,56.75));
#44550=CARTESIAN_POINT('',(-59.725,-52.425,56.75));
#44551=CARTESIAN_POINT('Origin',(-56.25,18.75,56.75));
#44552=CARTESIAN_POINT('',(-62.75,18.75,56.5));
#44553=CARTESIAN_POINT('',(-63.,18.75,56.75));
#44554=CARTESIAN_POINT('Origin',(-56.25,18.75,56.5));
#44555=CARTESIAN_POINT('Origin',(-56.25,18.75,57.));
#44556=CARTESIAN_POINT('',(-62.75,18.75,57.));
#44557=CARTESIAN_POINT('Origin',(-18.75,56.25,56.75));
#44558=CARTESIAN_POINT('',(-25.25,56.25,56.5));
#44559=CARTESIAN_POINT('',(-25.5,56.25,56.75));
#44560=CARTESIAN_POINT('Origin',(-18.75,56.25,56.5));
#44561=CARTESIAN_POINT('Origin',(-18.75,56.25,57.));
#44562=CARTESIAN_POINT('',(-25.25,56.25,57.));
#44563=CARTESIAN_POINT('Origin',(-52.425,52.425,42.75));
#44564=CARTESIAN_POINT('',(-56.6629,52.425,42.75));
#44565=CARTESIAN_POINT('Origin',(-85.725,-85.725,42.75));
#82346=UNCERTAINTY_MEASURE_WITH_UNIT(LENGTH_MEASURE(0.01),#82385,
'DISTANCE_ACCURACY_VALUE',
'Maximum model space distance between geometric entities at asserted c
onnectivities');
#82363=UNCERTAINTY_MEASURE_WITH_UNIT(LENGTH_MEASURE(0.01),#82385,
'DISTANCE_ACCURACY_VALUE',
'Maximum model space distance between geometric entities at asserted c
onnectivities');
#82367=(
GEOMETRIC_REPRESENTATION_CONTEXT(3)
GLOBAL_UNCERTAINTY_ASSIGNED_CONTEXT((#82346))
GLOBAL_UNIT_ASSIGNED_CONTEXT((#82385,#82387,#82388))
REPRESENTATION_CONTEXT('','3D')
);
#82384=(
GEOMETRIC_REPRESENTATION_CONTEXT(3)
GLOBAL_UNCERTAINTY_ASSIGNED_CONTEXT((#82363))
GLOBAL_UNIT_ASSIGNED_CONTEXT((#82385,#82387,#82388))
REPRESENTATION_CONTEXT('','3D')
);
#82385=(
LENGTH_UNIT()
NAMED_UNIT(*)
SI_UNIT(.MILLI.,.METRE.)
);
#82387=(
NAMED_UNIT(*)
PLANE_ANGLE_UNIT()
SI_UNIT($,.RADIAN.)
);
#82388=(
NAMED_UNIT(*)
SI_UNIT($,.STERADIAN.)
SOLID_ANGLE_UNIT()
);
#82392=SHAPE_DEFINITION_REPRESENTATION(#82412,#82468);
#82412=PRODUCT_DEFINITION_SHAPE('',$,#82489);
#82468=SHAPE_REPRESENTATION('',(#31321),#82367);
#82485=PRODUCT_DEFINITION_CONTEXT('part definition',#82547,'design');
#82489=PRODUCT_DEFINITION('2026-10-20-12-38-07-933',
'03_Top_Tilt_Platform',#82509,#82485);
#82509=PRODUCT_DEFINITION_FORMATION('',$,#82552);
#82547=APPLICATION_CONTEXT(
'Core Data for Automotive Mechanical Design Process');
#82548=PRODUCT_CONTEXT('part definition',#82547,'mechanical');
#82552=PRODUCT('2026-10-20-12-38-07-933','03_Top_Tilt_Platform',$,(#82548));
#82639=COLOUR_RGB('Off White',0.89,0.88,0.83);
#82640=FILL_AREA_STYLE_COLOUR('',#82639);
#82641=FILL_AREA_STYLE('',(#82640));
#82642=SURFACE_STYLE_FILL_AREA(#82641);
#82643=SURFACE_SIDE_STYLE('',(#82642));
#82644=SURFACE_STYLE_USAGE(.BOTH.,#82643);
#82645=PRESENTATION_STYLE_ASSIGNMENT((#82644));
ENDSEC;
END-ISO-10303-21;
